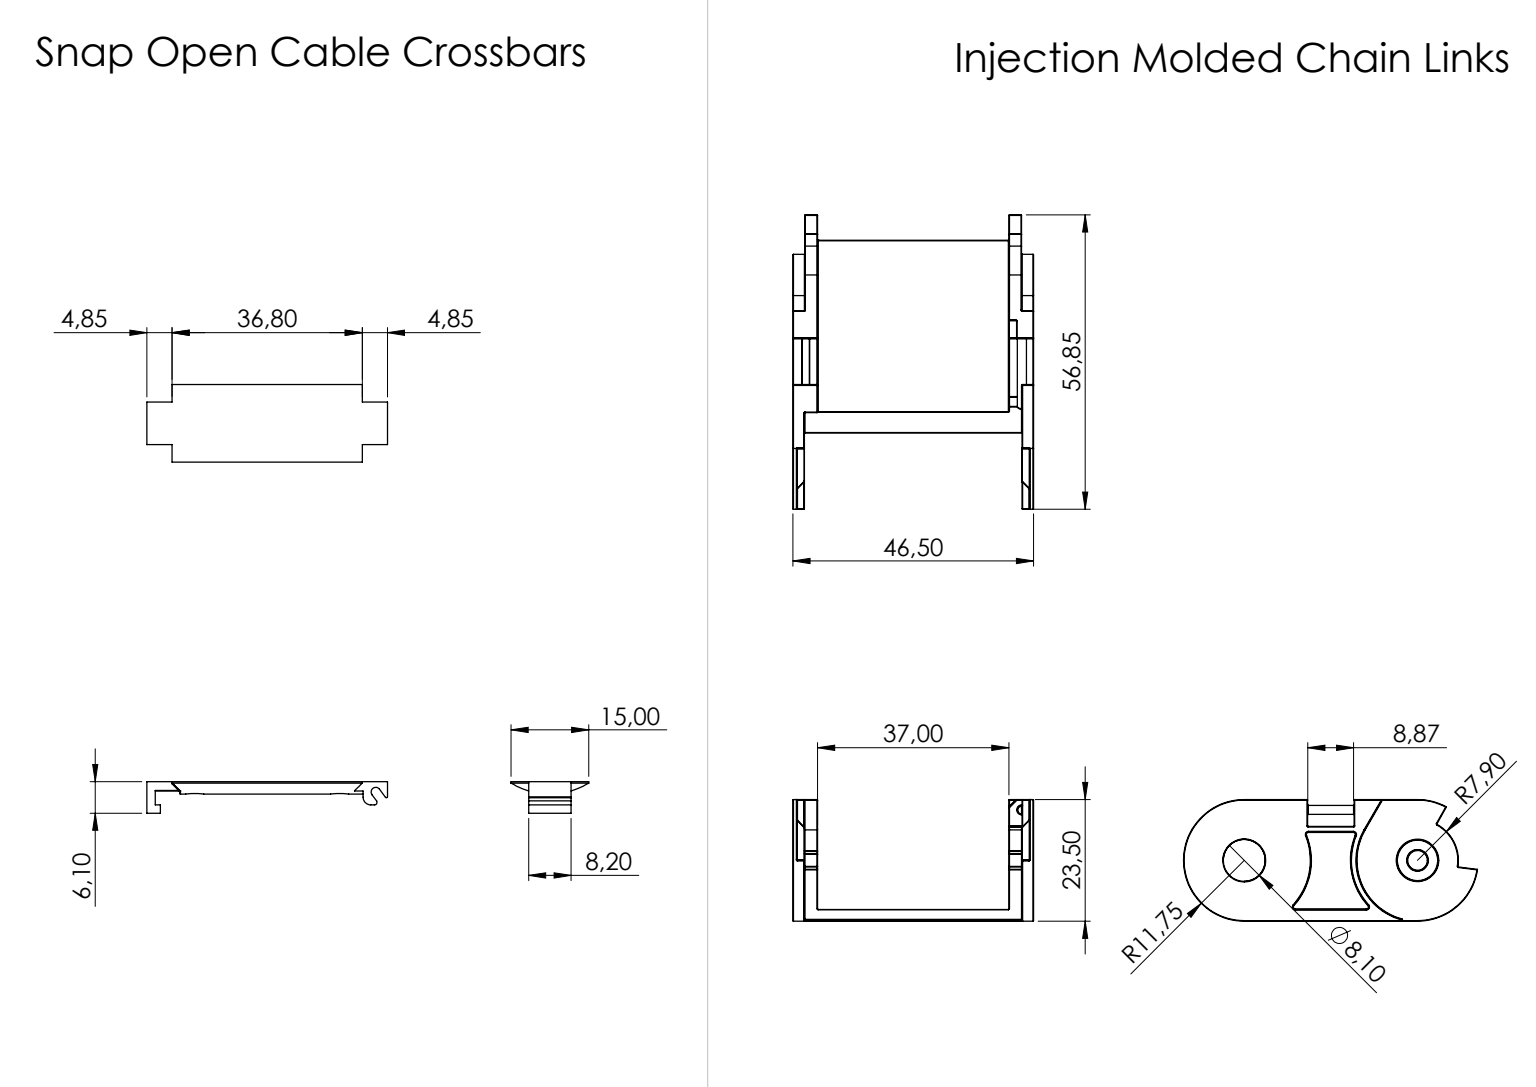
ISO-10303-21;
HEADER;
FILE_DESCRIPTION (('STEP AP214'),
    '1' );
FILE_NAME ('Snap Open Cable Crossbars.step',
    '2026-10-08T22:59:04',
    ( '' ),
    ( '' ),
    'SwSTEP 2.0',
    'SolidWorks 2020',
    '' );
FILE_SCHEMA (( 'AUTOMOTIVE_DESIGN' ));
ENDSEC;

DATA;
#1=CARTESIAN_POINT ( 'NONE',  ( -16.92989143108098204, 9.949999999999981526, -12.88248387475667656 ) ) ;
#36=CARTESIAN_POINT ( 'NONE',  ( -17.29838795458766043, 10.37154985795013218, -11.39525871738185714 ) ) ;
#202=CARTESIAN_POINT ( 'NONE',  ( 20.99999999999999645, 9.749999999999982236, -9.250000000000001776 ) ) ;
#413=CYLINDRICAL_SURFACE ( 'NONE', #45294, 1.749999999999998002 ) ;
#816=VERTEX_POINT ( 'NONE', #22856 ) ;
#827=FACE_OUTER_BOUND ( 'NONE', #190311, .T. ) ;
#850=CARTESIAN_POINT ( 'NONE',  ( -16.89797118371581419, 9.976380722644179855, -12.56270663244076857 ) ) ;
#880=FACE_OUTER_BOUND ( 'NONE', #179454, .T. ) ;
#1084=EDGE_CURVE ( 'NONE', #166202, #45065, #38658, .T. ) ;
#1259=CARTESIAN_POINT ( 'NONE',  ( -12.33960340485503515, 9.360749169915104417, -17.31457014060726962 ) ) ;
#1268=EDGE_CURVE ( 'NONE', #177395, #152802, #103725, .T. ) ;
#1311=DIRECTION ( 'NONE',  ( 1.000000000000000000, 0.000000000000000000, 0.000000000000000000 ) ) ;
#1354=ADVANCED_FACE ( 'NONE', ( #88580 ), #208179, .T. ) ;
#1447=DIRECTION ( 'NONE',  ( 1.652117596168391700E-15, 1.000000000000000000, -0.000000000000000000 ) ) ;
#1682=EDGE_CURVE ( 'NONE', #64185, #88756, #170443, .T. ) ;
#2076=AXIS2_PLACEMENT_3D ( 'NONE', #145577, #223822, #26957 ) ;
#2425=AXIS2_PLACEMENT_3D ( 'NONE', #153513, #135160, #16531 ) ;
#2428=ORIENTED_EDGE ( 'NONE', *, *, #175814, .F. ) ;
#2434=CARTESIAN_POINT ( 'NONE',  ( -16.94445028196807002, 9.992063609697737547, -20.89266982158155628 ) ) ;
#2476=APPLICATION_CONTEXT ( 'automotive_design' ) ;
#2634=CARTESIAN_POINT ( 'NONE',  ( -16.97683809663752186, 9.949999999999983302, -9.250000000000001776 ) ) ;
#2765=CARTESIAN_POINT ( 'NONE',  ( -17.78241384942186087, 10.85557575278904352, -23.25096232753543646 ) ) ;
#2813=EDGE_LOOP ( 'NONE', ( #157991, #36685, #88276, #78622 ) ) ;
#2957=FACE_OUTER_BOUND ( 'NONE', #112372, .T. ) ;
#3084=VECTOR ( 'NONE', #229687, 1000.000000000000000 ) ;
#3180=CARTESIAN_POINT ( 'NONE',  ( -16.80100914604134488, 9.943149094103565844, -20.81704412728764453 ) ) ;
#3672=ORIENTED_EDGE ( 'NONE', *, *, #139542, .F. ) ;
#4041=CARTESIAN_POINT ( 'NONE',  ( -12.47155713865592119, 9.375669526425772560, -15.86779000938594031 ) ) ;
#4143=DIRECTION ( 'NONE',  ( 1.186688945009009831E-16, -1.000000000000000000, 0.000000000000000000 ) ) ;
#4327=CARTESIAN_POINT ( 'NONE',  ( -23.25000000000000355, 5.649999999999983480, -12.65000000000000213 ) ) ;
#4347=FACE_OUTER_BOUND ( 'NONE', #98803, .T. ) ;
#4390=( BOUNDED_CURVE ( )  B_SPLINE_CURVE ( 3, ( #73328, #206387, #207681, #32928 ),
 .UNSPECIFIED., .F., .F. ) 
 B_SPLINE_CURVE_WITH_KNOTS ( ( 4, 4 ),
 ( 1.570796326794908992, 2.617993877991502849 ),
 .UNSPECIFIED. ) 
 CURVE ( )  GEOMETRIC_REPRESENTATION_ITEM ( )  RATIONAL_B_SPLINE_CURVE ( ( 1.000000000000000000, 0.9106836025229597675, 0.9106836025229597675, 1.000000000000000000 ) ) 
 REPRESENTATION_ITEM ( '' )  );
#4466=CARTESIAN_POINT ( 'NONE',  ( 14.22916352759893499, 9.457410930290162554, -18.49991590874628500 ) ) ;
#4575=CARTESIAN_POINT ( 'NONE',  ( -17.01825945287481545, 9.949999999999983302, -20.75000000000000000 ) ) ;
#4760=CARTESIAN_POINT ( 'NONE',  ( 18.39999999999999503, 11.74999999999998224, -20.85000000000000142 ) ) ;
#4794=( BOUNDED_SURFACE ( )  B_SPLINE_SURFACE ( 3, 2, ( 
 ( #64703, #180813, #239501 ),
 ( #179541, #850, #161255 ),
 ( #122121, #63409, #201646 ),
 ( #139068, #120862, #98653 ) ),
 .UNSPECIFIED., .F., .F., .T. ) 
 B_SPLINE_SURFACE_WITH_KNOTS ( ( 4, 4 ),
 ( 3, 3 ),
 ( 0.0008258556059633813742, 0.0009616864997632797044 ),
 ( 0.000000000000000000, 1.000000000000000000 ),
 .UNSPECIFIED. ) 
 GEOMETRIC_REPRESENTATION_ITEM ( )  RATIONAL_B_SPLINE_SURFACE ( (
 ( 1.000000000000000000, 0.9152888060719355234, 1.000000000000000000),
 ( 1.000000000000000000, 0.9327727094138189567, 1.000000000000000000),
 ( 1.000000000000000000, 0.9369023509258441740, 1.000000000000000000),
 ( 1.000000000000000000, 0.9246339933864472505, 1.000000000000000000) ) ) 
 REPRESENTATION_ITEM ( '' )  SURFACE ( )  );
#4866=CARTESIAN_POINT ( 'NONE',  ( -16.87331047859651179, 9.949999999999986855, -12.65000000000000213 ) ) ;
#4911=CARTESIAN_POINT ( 'NONE',  ( -16.94878442675511465, 9.991729102990998257, -20.88821957563787635 ) ) ;
#4939=VECTOR ( 'NONE', #199116, 1000.000000000000000 ) ;
#4994=DIRECTION ( 'NONE',  ( 1.000000000000000000, 0.000000000000000000, 0.000000000000000000 ) ) ;
#5134=AXIS2_PLACEMENT_3D ( 'NONE', #210609, #250995, #127226 ) ;
#5409=VERTEX_POINT ( 'NONE', #97085 ) ;
#5553=CARTESIAN_POINT ( 'NONE',  ( 20.73486653747088226, 7.250000000000026645, -12.65000000000000568 ) ) ;
#5607=CARTESIAN_POINT ( 'NONE',  ( -16.89208623190940273, 9.951577948975481647, -20.85527220321827002 ) ) ;
#6030=FACE_OUTER_BOUND ( 'NONE', #166234, .T. ) ;
#6408=CARTESIAN_POINT ( 'NONE',  ( -12.60829076262180060, 9.389529397466734650, -17.81710791289367535 ) ) ;
#6428=PLANE ( 'NONE',  #186510 ) ;
#6469=AXIS2_PLACEMENT_3D ( 'NONE', #223394, #44779, #100847 ) ;
#6649=AXIS2_PLACEMENT_3D ( 'NONE', #142927, #174758, #96432 ) ;
#6857=DIRECTION ( 'NONE',  ( 0.5932847527679299127, -0.8049926720990051576, 6.366092712777055223E-16 ) ) ;
#6912=( NAMED_UNIT ( * ) SI_UNIT ( $, .STERADIAN. ) SOLID_ANGLE_UNIT ( ) );
#6991=ORIENTED_EDGE ( 'NONE', *, *, #49751, .F. ) ;
#7235=VERTEX_POINT ( 'NONE', #177601 ) ;
#7280=ADVANCED_FACE ( 'NONE', ( #99288 ), #178892, .F. ) ;
#7551=CARTESIAN_POINT ( 'NONE',  ( -16.87036670365548474, 10.08494996325527460, -20.94999999999999929 ) ) ;
#7806=FACE_OUTER_BOUND ( 'NONE', #23507, .T. ) ;
#7861=AXIS2_PLACEMENT_3D ( 'NONE', #232656, #11018, #53993 ) ;
#7969=VERTEX_POINT ( 'NONE', #147105 ) ;
#8041=DIRECTION ( 'NONE',  ( 0.000000000000000000, 0.000000000000000000, -1.000000000000000000 ) ) ;
#8080=DIRECTION ( 'NONE',  ( 1.000000000000000000, 0.000000000000000000, -0.000000000000000000 ) ) ;
#8152=ADVANCED_FACE ( 'NONE', ( #23040 ), #4794, .T. ) ;
#8294=CARTESIAN_POINT ( 'NONE',  ( -23.25000000000000355, 5.649999999999983480, -9.250000000000001776 ) ) ;
#8359=LINE ( 'NONE', #9625, #132434 ) ;
#8639=CARTESIAN_POINT ( 'NONE',  ( -16.93658623642901162, 9.980381671657131193, -12.61190272912918964 ) ) ;
#8647=FACE_OUTER_BOUND ( 'NONE', #161256, .T. ) ;
#8875=CARTESIAN_POINT ( 'NONE',  ( -16.86578989773640913, 9.984809801258796469, -20.96466488662223426 ) ) ;
#9058=AXIS2_PLACEMENT_3D ( 'NONE', #124611, #201562, #162464 ) ;
#9153=DIRECTION ( 'NONE',  ( 1.000000000000000000, -0.000000000000000000, -0.000000000000000000 ) ) ;
#9473=ORIENTED_EDGE ( 'NONE', *, *, #1084, .F. ) ;
#9625=CARTESIAN_POINT ( 'NONE',  ( -23.25000000000000355, 11.74999999999998224, -24.25000000000000000 ) ) ;
#9635=DIRECTION ( 'NONE',  ( -1.020425574104004196E-15, 0.000000000000000000, -1.000000000000000000 ) ) ;
#9814=DIRECTION ( 'NONE',  ( 0.000000000000000000, 1.000000000000000000, 3.662759245464225434E-15 ) ) ;
#9888=FACE_OUTER_BOUND ( 'NONE', #185101, .T. ) ;
#10255=CARTESIAN_POINT ( 'NONE',  ( -16.93226657140833069, 9.999543822724415776, -12.57871311097362188 ) ) ;
#10281=CARTESIAN_POINT ( 'NONE',  ( -15.51798037960205257, 9.376659938533535410, -17.62819254821728876 ) ) ;
#10503=CARTESIAN_POINT ( 'NONE',  ( -18.40000000000000213, 11.47316190336247388, -12.65000000000000213 ) ) ;
#10606=CARTESIAN_POINT ( 'NONE',  ( -17.11825945287482753, 10.04999999999998295, -12.65000000000000213 ) ) ;
#10621=ORIENTED_EDGE ( 'NONE', *, *, #251969, .F. ) ;
#10937=DIRECTION ( 'NONE',  ( 1.000000000000000000, 0.000000000000000000, -1.020425574104004196E-15 ) ) ;
#10962=CARTESIAN_POINT ( 'NONE',  ( -16.86133551771149541, 9.949999999999983302, -20.80134343454665213 ) ) ;
#10978=ORIENTED_EDGE ( 'NONE', *, *, #1268, .F. ) ;
#11018=DIRECTION ( 'NONE',  ( 1.186688945009009831E-16, -1.000000000000000000, 0.000000000000000000 ) ) ;
#11145=CYLINDRICAL_SURFACE ( 'NONE', #172793, 0.1999999999999987899 ) ;
#11416=VECTOR ( 'NONE', #214106, 1000.000000000000000 ) ;
#11464=ORIENTED_EDGE ( 'NONE', *, *, #189871, .T. ) ;
#11901=LINE ( 'NONE', #189239, #247679 ) ;
#11925=AXIS2_PLACEMENT_3D ( 'NONE', #48197, #126453, #143448 ) ;
#12016=LINE ( 'NONE', #69418, #173208 ) ;
#12179=( BOUNDED_CURVE ( )  B_SPLINE_CURVE ( 3, ( #253467, #111406, #110112, #74881 ),
 .UNSPECIFIED., .F., .T. ) 
 B_SPLINE_CURVE_WITH_KNOTS ( ( 4, 4 ),
 ( 0.3000847527772381174, 0.5497968875596821459 ),
 .UNSPECIFIED. ) 
 CURVE ( )  GEOMETRIC_REPRESENTATION_ITEM ( )  RATIONAL_B_SPLINE_CURVE ( ( 1.000000000000000000, 0.9948104011409419911, 0.9948104011409419911, 1.000000000000000000 ) ) 
 REPRESENTATION_ITEM ( '' )  );
#12209=CARTESIAN_POINT ( 'NONE',  ( 13.22461703343584638, 9.436662931799084220, -18.32303673229488794 ) ) ;
#12294=CARTESIAN_POINT ( 'NONE',  ( 18.39999999999999503, 11.74999999999998224, -12.65000000000000213 ) ) ;
#12434=FACE_OUTER_BOUND ( 'NONE', #157664, .T. ) ;
#12804=DIRECTION ( 'NONE',  ( -1.000000000000000000, 1.652117596168391700E-15, 0.000000000000000000 ) ) ;
#12859=VECTOR ( 'NONE', #213521, 1000.000000000000000 ) ;
#12920=VERTEX_POINT ( 'NONE', #158155 ) ;
#12996=EDGE_LOOP ( 'NONE', ( #33480, #208453, #194883, #57495 ) ) ;
#13020=EDGE_CURVE ( 'NONE', #33881, #237173, #25040, .T. ) ;
#13083=VECTOR ( 'NONE', #54298, 1000.000000000000000 ) ;
#13218=DIRECTION ( 'NONE',  ( -0.5932847527679310229, 0.8049926720990042694, -6.366092712777067056E-16 ) ) ;
#13289=VECTOR ( 'NONE', #57030, 1000.000000000000000 ) ;
#13474=CARTESIAN_POINT ( 'NONE',  ( -16.77431908686106610, 9.945805754517978770, -12.66416078234975373 ) ) ;
#13481=CARTESIAN_POINT ( 'NONE',  ( 13.12229106158772929, 9.430637101696738966, -18.26826061806094614 ) ) ;
#13689=CARTESIAN_POINT ( 'NONE',  ( 12.25000000000000000, 9.349999999999983658, -16.74999999999999645 ) ) ;
#13778=FACE_OUTER_BOUND ( 'NONE', #117729, .T. ) ;
#13843=DIRECTION ( 'NONE',  ( -1.000000000000000000, 0.000000000000000000, -0.000000000000000000 ) ) ;
#13882=VECTOR ( 'NONE', #129686, 1000.000000000000000 ) ;
#14008=( LENGTH_UNIT ( ) NAMED_UNIT ( * ) SI_UNIT ( .MILLI., .METRE. ) );
#14057=AXIS2_PLACEMENT_3D ( 'NONE', #196592, #214877, #97468 ) ;
#14206=CARTESIAN_POINT ( 'NONE',  ( 20.73486653747090003, 7.250000000000026645, -20.85000000000000142 ) ) ;
#14615=VERTEX_POINT ( 'NONE', #34702 ) ;
#14701=ORIENTED_EDGE ( 'NONE', *, *, #49751, .T. ) ;
#14727=CARTESIAN_POINT ( 'NONE',  ( -16.94275863006528482, 9.989496048667513506, -20.89169738207657900 ) ) ;
#14735=CARTESIAN_POINT ( 'NONE',  ( -16.77683809663752257, 23.65833333333332433, -16.75000000000000000 ) ) ;
#15047=CARTESIAN_POINT ( 'NONE',  ( -18.35235881385853318, 11.47341900771289502, -9.250000000000001776 ) ) ;
#15165=PLANE ( 'NONE',  #223421 ) ;
#15643=ADVANCED_FACE ( 'NONE', ( #217183 ), #15165, .T. ) ;
#15874=ORIENTED_EDGE ( 'NONE', *, *, #175580, .T. ) ;
#15938=CARTESIAN_POINT ( 'NONE',  ( 23.04999999999999716, 8.822561741666397950, -12.65000000000000746 ) ) ;
#15952=CYLINDRICAL_SURFACE ( 'NONE', #238205, 0.1000000000000001443 ) ;
#16009=CARTESIAN_POINT ( 'NONE',  ( -16.93301857435212554, 9.976309354735457546, -20.88577557116142813 ) ) ;
#16028=CARTESIAN_POINT ( 'NONE',  ( -16.87036670365548474, 9.989418819301645769, -20.97956011730205006 ) ) ;
#16220=DIRECTION ( 'NONE',  ( -1.000000000000000000, -0.000000000000000000, 1.073024830501117725E-15 ) ) ;
#16242=CIRCLE ( 'NONE', #7861, 1.749999999999998002 ) ;
#16369=VECTOR ( 'NONE', #222084, 1000.000000000000000 ) ;
#16512=CARTESIAN_POINT ( 'NONE',  ( -16.93826681692523195, 10.01142872028771258, -20.94545846735944039 ) ) ;
#16531=DIRECTION ( 'NONE',  ( 1.000000000000000000, 0.000000000000000000, 0.000000000000000000 ) ) ;
#16707=EDGE_CURVE ( 'NONE', #101212, #219433, #149599, .T. ) ;
#16728=EDGE_LOOP ( 'NONE', ( #255760, #202446, #84176, #145665, #190088, #218155 ) ) ;
#16867=VECTOR ( 'NONE', #108313, 1000.000000000000000 ) ;
#16914=ORIENTED_EDGE ( 'NONE', *, *, #147422, .F. ) ;
#17161=VERTEX_POINT ( 'NONE', #4327 ) ;
#17354=CARTESIAN_POINT ( 'NONE',  ( -16.77683809663752257, 9.945835743204147761, -20.83605098089580210 ) ) ;
#17399=EDGE_CURVE ( 'NONE', #195135, #51112, #36791, .T. ) ;
#17460=( BOUNDED_CURVE ( )  B_SPLINE_CURVE ( 3, ( #10606, #90112, #169715, #191834 ),
 .UNSPECIFIED., .F., .F. ) 
 B_SPLINE_CURVE_WITH_KNOTS ( ( 4, 4 ),
 ( 4.712388980384689674, 5.672655318024675708 ),
 .UNSPECIFIED. ) 
 CURVE ( )  GEOMETRIC_REPRESENTATION_ITEM ( )  RATIONAL_B_SPLINE_CURVE ( ( 1.000000000000000000, 0.9246222802177378464, 0.9246222802177378464, 1.000000000000000000 ) ) 
 REPRESENTATION_ITEM ( '' )  );
#17529=CARTESIAN_POINT ( 'NONE',  ( 14.56326696814971555, 9.446648990628860432, -15.08916329592317851 ) ) ;
#17932=DIRECTION ( 'NONE',  ( -1.186688945009010077E-16, 1.000000000000000000, 0.000000000000000000 ) ) ;
#17968=CARTESIAN_POINT ( 'NONE',  ( -20.65000000000000568, 7.249999999999983125, -9.250000000000001776 ) ) ;
#18030=VERTEX_POINT ( 'NONE', #147078 ) ;
#18241=PRODUCT_CONTEXT ( 'NONE', #208885, 'mechanical' ) ;
#18310=CARTESIAN_POINT ( 'NONE',  ( -23.25000000000000355, 5.649999999999983480, -9.250000000000001776 ) ) ;
#18323=FACE_OUTER_BOUND ( 'NONE', #43596, .T. ) ;
#18823=CARTESIAN_POINT ( 'NONE',  ( 15.74999999999999645, 9.349999999999983658, -16.75000000000000000 ) ) ;
#18974=CARTESIAN_POINT ( 'NONE',  ( -18.40000000000000213, 5.649999999999983480, -12.65000000000000213 ) ) ;
#19226=DIRECTION ( 'NONE',  ( 1.000000000000000000, 1.186688945009010077E-16, 0.000000000000000000 ) ) ;
#19555=LINE ( 'NONE', #219015, #142994 ) ;
#19583=ORIENTED_EDGE ( 'NONE', *, *, #49360, .F. ) ;
#19621=CARTESIAN_POINT ( 'NONE',  ( -17.22767730082987825, 10.34924421246758719, -11.35757130942880977 ) ) ;
#19659=EDGE_LOOP ( 'NONE', ( #155323, #54902, #200500, #42750 ) ) ;
#19983=AXIS2_PLACEMENT_3D ( 'NONE', #126963, #206498, #82661 ) ;
#20072=CARTESIAN_POINT ( 'NONE',  ( -23.25000000000000355, 11.74999999999998224, -12.65000000000000213 ) ) ;
#20073=SURFACE_STYLE_FILL_AREA ( #120478 ) ;
#20155=ADVANCED_FACE ( 'NONE', ( #147502 ), #167102, .F. ) ;
#20208=CARTESIAN_POINT ( 'NONE',  ( -16.87683809663752044, 9.864913447280185821, -20.22428155130396021 ) ) ;
#20381=ORIENTED_EDGE ( 'NONE', *, *, #229317, .F. ) ;
#20491=FACE_OUTER_BOUND ( 'NONE', #166229, .T. ) ;
#20500=AXIS2_PLACEMENT_3D ( 'NONE', #162836, #4994, #63705 ) ;
#20521=ORIENTED_EDGE ( 'NONE', *, *, #17399, .F. ) ;
#20595=EDGE_CURVE ( 'NONE', #35963, #143544, #181618, .T. ) ;
#21033=CARTESIAN_POINT ( 'NONE',  ( -16.97683809663752186, 9.949999999999983302, -13.40236401819648648 ) ) ;
#21051=CARTESIAN_POINT ( 'NONE',  ( -21.64999999999999858, 9.349999999999978328, -20.85000000000000142 ) ) ;
#21147=CARTESIAN_POINT ( 'NONE',  ( -33.72168855820452649, 11.47316190336247033, -9.249999999999998224 ) ) ;
#21154=EDGE_CURVE ( 'NONE', #7969, #237173, #245177, .T. ) ;
#21199=VECTOR ( 'NONE', #124420, 1000.000000000000000 ) ;
#21286=ORIENTED_EDGE ( 'NONE', *, *, #159207, .F. ) ;
#21319=PLANE ( 'NONE',  #241824 ) ;
#21353=EDGE_CURVE ( 'NONE', #101212, #222175, #16242, .T. ) ;
#21382=EDGE_CURVE ( 'NONE', #60760, #177395, #12179, .T. ) ;
#21496=CARTESIAN_POINT ( 'NONE',  ( -16.88705144915421030, 9.949999999999981526, -20.56902140528771739 ) ) ;
#21501=CARTESIAN_POINT ( 'NONE',  ( -16.81453563122428818, 9.939100205436954383, -20.78825866064531880 ) ) ;
#21515=CARTESIAN_POINT ( 'NONE',  ( 18.39999999999999503, 11.74999999999998224, -20.85000000000000142 ) ) ;
#21775=DIRECTION ( 'NONE',  ( -0.7071067811865487940, 0.7071067811865463515, 0.000000000000000000 ) ) ;
#21962=EDGE_LOOP ( 'NONE', ( #16914, #90521, #72160, #246736 ) ) ;
#22093=CARTESIAN_POINT ( 'NONE',  ( 20.99999999999999645, 9.749999999999982236, -12.65000000000000568 ) ) ;
#22353=CARTESIAN_POINT ( 'NONE',  ( -12.84409460144754433, 9.410682294267951775, -15.43114344194827581 ) ) ;
#22370=CARTESIAN_POINT ( 'NONE',  ( -16.91256925476569961, 9.985731158128169582, -20.96764248900526439 ) ) ;
#22621=B_SPLINE_CURVE_WITH_KNOTS ( 'NONE', 3,
 ( #154744, #16512, #93447, #173048, #153491, #135134, #36070, #232999, #214684, #195162, #96013, #255032, #129999, #209563, #30956, #170489 ),
 .UNSPECIFIED., .F., .F.,
 ( 4, 3, 3, 3, 3, 4 ),
 ( 0.000000000000000000, 1.810570668010556722E-05, 2.740575833571567380E-05, 4.256816319435758028E-05, 5.213463471025523268E-05, 6.641585710718234082E-05 ),
 .UNSPECIFIED. ) ;
#22712=( BOUNDED_CURVE ( )  B_SPLINE_CURVE ( 3, ( #227470, #48840, #207945, #192227 ),
 .UNSPECIFIED., .F., .F. ) 
 B_SPLINE_CURVE_WITH_KNOTS ( ( 4, 4 ),
 ( 1.570796326794885012, 3.141592653589794448 ),
 .UNSPECIFIED. ) 
 CURVE ( )  GEOMETRIC_REPRESENTATION_ITEM ( )  RATIONAL_B_SPLINE_CURVE ( ( 1.000000000000000000, 0.8047378541243619399, 0.8047378541243619399, 1.000000000000000000 ) ) 
 REPRESENTATION_ITEM ( '' )  );
#22727=EDGE_CURVE ( 'NONE', #203977, #5409, #248862, .T. ) ;
#22788=CARTESIAN_POINT ( 'NONE',  ( -16.84793658983420173, 9.949999999999983302, -20.76635332218982910 ) ) ;
#22795=CARTESIAN_POINT ( 'NONE',  ( -16.80469485234340610, 9.942151663141038043, -20.80996684393117135 ) ) ;
#22856=CARTESIAN_POINT ( 'NONE',  ( -17.11825945287482753, 10.04999999999998295, -12.65000000000000213 ) ) ;
#23040=FACE_OUTER_BOUND ( 'NONE', #19659, .T. ) ;
#23258=CARTESIAN_POINT ( 'NONE',  ( -20.65000000000000568, 5.649999999999983480, -9.250000000000001776 ) ) ;
#23445=CARTESIAN_POINT ( 'NONE',  ( -14.77538296656415184, 9.436662931799085996, -18.32303673229489149 ) ) ;
#23507=EDGE_LOOP ( 'NONE', ( #57717, #253160, #179128, #59181 ) ) ;
#23649=CARTESIAN_POINT ( 'NONE',  ( -15.06774609480955363, 9.417651958841000592, -15.35878739244043345 ) ) ;
#23659=CARTESIAN_POINT ( 'NONE',  ( 18.39999999999999147, 8.822561741666397950, -9.250000000000001776 ) ) ;
#23666=CARTESIAN_POINT ( 'NONE',  ( -18.41431012584568805, 11.48747202920817223, -24.27323601310168399 ) ) ;
#23835=ORIENTED_EDGE ( 'NONE', *, *, #81866, .F. ) ;
#23843=CARTESIAN_POINT ( 'NONE',  ( -23.25000000000000355, 5.649999999999983480, -20.85000000000000142 ) ) ;
#23960=PLANE ( 'NONE',  #112128 ) ;
#24301=CARTESIAN_POINT ( 'NONE',  ( -16.87036670365549895, 10.08494996325527460, -12.55000000000000249 ) ) ;
#24387=DIRECTION ( 'NONE',  ( 1.000000000000000000, -0.000000000000000000, -0.000000000000000000 ) ) ;
#24490=CARTESIAN_POINT ( 'NONE',  ( -16.89060415895971090, 9.951220762802197584, -12.64592022427046203 ) ) ;
#24938=EDGE_CURVE ( 'NONE', #187424, #206683, #225373, .T. ) ;
#25035=EDGE_CURVE ( 'NONE', #195135, #201670, #188355, .T. ) ;
#25040=LINE ( 'NONE', #182832, #147141 ) ;
#25053=DIRECTION ( 'NONE',  ( 1.000000000000000000, 0.000000000000000000, -0.000000000000000000 ) ) ;
#25524=ORIENTED_EDGE ( 'NONE', *, *, #180090, .T. ) ;
#25572=CARTESIAN_POINT ( 'NONE',  ( 20.73486653747088937, 7.750000000000025757, -9.250000000000001776 ) ) ;
#25783=CYLINDRICAL_SURFACE ( 'NONE', #213675, 1.500000000000001332 ) ;
#25802=ORIENTED_EDGE ( 'NONE', *, *, #247500, .T. ) ;
#25834=DIRECTION ( 'NONE',  ( 1.000000000000000000, -0.000000000000000000, -0.000000000000000000 ) ) ;
#25989=CARTESIAN_POINT ( 'NONE',  ( -12.30589683808040391, 9.356746017078247490, -17.20335972136419400 ) ) ;
#26607=CARTESIAN_POINT ( 'NONE',  ( -15.75000000000000355, 9.849999999999978328, -16.75000000000000355 ) ) ;
#26839=CARTESIAN_POINT ( 'NONE',  ( -17.29158576265543346, 10.36474766601791586, -22.08275824479217775 ) ) ;
#26957=DIRECTION ( 'NONE',  ( 0.000000000000000000, 0.000000000000000000, 1.000000000000000000 ) ) ;
#27150=CARTESIAN_POINT ( 'NONE',  ( 20.73486653747088582, 7.250000000000026645, -9.250000000000001776 ) ) ;
#27284=FACE_BOUND ( 'NONE', #27743, .T. ) ;
#27305=VECTOR ( 'NONE', #238398, 1000.000000000000000 ) ;
#27497=VECTOR ( 'NONE', #66820, 1000.000000000000000 ) ;
#27743=EDGE_LOOP ( 'NONE', ( #45441, #134007 ) ) ;
#27882=ADVANCED_FACE ( 'NONE', ( #30508 ), #188274, .F. ) ;
#27978=VERTEX_POINT ( 'NONE', #17354 ) ;
#28030=( BOUNDED_SURFACE ( )  B_SPLINE_SURFACE ( 3, 2, ( 
 ( #249522, #52578, #33078 ),
 ( #173875, #53880, #74764 ),
 ( #55123, #154311, #168742 ),
 ( #70901, #134672, #209094 ),
 ( #248228, #69603, #149146 ),
 ( #229942, #228680, #91719 ),
 ( #30478, #112577, #252071 ),
 ( #51271, #250784, #31779 ),
 ( #111287, #171311, #151725 ),
 ( #231252, #192126, #13474 ) ),
 .UNSPECIFIED., .F., .F., .F. ) 
 B_SPLINE_SURFACE_WITH_KNOTS ( ( 4, 2, 2, 2, 4 ),
 ( 3, 3 ),
 ( 0.002161241639767788603, 0.002579950749617449836, 0.002789305304542280452, 0.002893982582004695978, 0.002998659859467111069 ),
 ( 0.000000000000000000, 1.000000000000000000 ),
 .UNSPECIFIED. ) 
 GEOMETRIC_REPRESENTATION_ITEM ( )  RATIONAL_B_SPLINE_SURFACE ( (
 ( 1.000000000000000000, 0.7071067811864800712, 1.000000000000000000),
 ( 1.000000000000000000, 0.7632447400664645887, 1.000000000000000000),
 ( 1.000000000000000000, 0.8158073005108372744, 1.000000000000000000),
 ( 1.000000000000000000, 0.8906973462396270413, 1.000000000000000000),
 ( 1.000000000000000000, 0.9149408947800815595, 1.000000000000000000),
 ( 1.000000000000000000, 0.9493368785275272392, 1.000000000000000000),
 ( 1.000000000000000000, 0.9605194247156589871, 1.000000000000000000),
 ( 1.000000000000000000, 0.9803630264781161285, 1.000000000000000000),
 ( 1.000000000000000000, 0.9900844824271106681, 1.000000000000000000),
 ( 1.000000000000000000, 0.9894588281429282928, 1.000000000000000000) ) ) 
 REPRESENTATION_ITEM ( '' )  SURFACE ( )  );
#28151=PLANE ( 'NONE',  #5134 ) ;
#28343=PLANE ( 'NONE',  #214509 ) ;
#28391=DIRECTION ( 'NONE',  ( -0.000000000000000000, -0.000000000000000000, -1.000000000000000000 ) ) ;
#28480=CARTESIAN_POINT ( 'NONE',  ( -16.86337532320260735, 9.979967204224358568, -20.94892446898280980 ) ) ;
#28482=CYLINDRICAL_SURFACE ( 'NONE', #20500, 0.09999999999999939493 ) ;
#28535=VECTOR ( 'NONE', #219008, 1000.000000000000000 ) ;
#28727=EDGE_CURVE ( 'NONE', #184131, #86042, #85956, .T. ) ;
#28914=VECTOR ( 'NONE', #211018, 999.9999999999998863 ) ;
#28990=VERTEX_POINT ( 'NONE', #206590 ) ;
#29224=CARTESIAN_POINT ( 'NONE',  ( 15.31784899511109721, 9.396630376317714806, -17.90705739281830589 ) ) ;
#29249=CARTESIAN_POINT ( 'NONE',  ( -18.40000000000000213, 5.649999999999983480, -12.65000000000000213 ) ) ;
#29270=ORIENTED_EDGE ( 'NONE', *, *, #21154, .F. ) ;
#29462=CARTESIAN_POINT ( 'NONE',  ( 13.99999999999999822, 9.849999999999981881, -16.74999999999999645 ) ) ;
#29712=DIRECTION ( 'NONE',  ( -0.000000000000000000, -0.000000000000000000, -1.000000000000000000 ) ) ;
#29737=EDGE_CURVE ( 'NONE', #109071, #191176, #181304, .T. ) ;
#29931=ORIENTED_EDGE ( 'NONE', *, *, #35996, .T. ) ;
#30247=VECTOR ( 'NONE', #92407, 1000.000000000000000 ) ;
#30478=CARTESIAN_POINT ( 'NONE',  ( -16.87401514999235630, 9.949999999999983302, -12.71998200746783780 ) ) ;
#30485=CARTESIAN_POINT ( 'NONE',  ( -16.77180007708460963, 9.949999999999983302, -20.86438588104518388 ) ) ;
#30508=FACE_OUTER_BOUND ( 'NONE', #227736, .T. ) ;
#30956=CARTESIAN_POINT ( 'NONE',  ( -16.94132844910801694, 9.992436755180344576, -20.89620175598231455 ) ) ;
#31003=ORIENTED_EDGE ( 'NONE', *, *, #159207, .T. ) ;
#31041=CARTESIAN_POINT ( 'NONE',  ( -16.86420534634261514, 9.970615445591718640, -20.91833654923738806 ) ) ;
#31064=CARTESIAN_POINT ( 'NONE',  ( -16.77683809663752257, 9.949999999999983302, -20.85000000000000142 ) ) ;
#31779=CARTESIAN_POINT ( 'NONE',  ( -16.80621392010906945, 9.942202577507719852, -12.68959196541704060 ) ) ;
#31835=CARTESIAN_POINT ( 'NONE',  ( -16.97683809663752186, 9.949999999999983302, -20.09763598180368405 ) ) ;
#31863=LINE ( 'NONE', #12294, #204867 ) ;
#32013=DIRECTION ( 'NONE',  ( -1.000000000000000000, 0.000000000000000000, 0.000000000000000000 ) ) ;
#32597=CIRCLE ( 'NONE', #86689, 1.749999999999999778 ) ;
#32808=CARTESIAN_POINT ( 'NONE',  ( 20.27550659511089037, 9.216043722508839409, -20.85000000000000142 ) ) ;
#32836=VECTOR ( 'NONE', #178947, 1000.000000000000000 ) ;
#32846=EDGE_CURVE ( 'NONE', #140173, #47344, #174568, .T. ) ;
#32855=ORIENTED_EDGE ( 'NONE', *, *, #46103, .F. ) ;
#32863=ORIENTED_EDGE ( 'NONE', *, *, #139800, .F. ) ;
#32911=CARTESIAN_POINT ( 'NONE',  ( -15.55912972643740488, 8.490870273562565629, -20.85000000000000142 ) ) ;
#32928=CARTESIAN_POINT ( 'NONE',  ( -16.87331047859649757, 9.949999999999983302, -20.85000000000000142 ) ) ;
#32958=DIRECTION ( 'NONE',  ( 0.7071067811865463515, -0.7071067811865487940, 0.000000000000000000 ) ) ;
#33016=CARTESIAN_POINT ( 'NONE',  ( -17.04295772865485148, 10.02489942525999567, -20.85000000000000142 ) ) ;
#33078=CARTESIAN_POINT ( 'NONE',  ( -16.87683809663752399, 9.849999999999964118, -13.40236401819648115 ) ) ;
#33275=CARTESIAN_POINT ( 'NONE',  ( -16.87683809663752399, 23.65833333333332433, -16.75000000000000000 ) ) ;
#33326=DIRECTION ( 'NONE',  ( -0.000000000000000000, -0.000000000000000000, -1.000000000000000000 ) ) ;
#33379=DIRECTION ( 'NONE',  ( 0.000000000000000000, 0.000000000000000000, 1.000000000000000000 ) ) ;
#33480=ORIENTED_EDGE ( 'NONE', *, *, #182872, .T. ) ;
#33583=CARTESIAN_POINT ( 'NONE',  ( -21.65000000000000213, 7.249999999999983125, -20.85000000000000142 ) ) ;
#33644=DIRECTION ( 'NONE',  ( -1.000000000000000000, 0.000000000000000000, 0.000000000000000000 ) ) ;
#33881=VERTEX_POINT ( 'NONE', #38907 ) ;
#34232=ORIENTED_EDGE ( 'NONE', *, *, #81714, .F. ) ;
#34413=CARTESIAN_POINT ( 'NONE',  ( 20.99999999999999645, 9.749999999999982236, -20.84999999999999787 ) ) ;
#34561=CARTESIAN_POINT ( 'NONE',  ( 15.52844286134407703, 9.375669526425774336, -15.86779000938593676 ) ) ;
#34650=DIRECTION ( 'NONE',  ( -1.073024830501117725E-15, -0.000000000000000000, -1.000000000000000000 ) ) ;
#34702=CARTESIAN_POINT ( 'NONE',  ( 22.88900146558018989, 8.703904791112817563, -20.84999999999999432 ) ) ;
#34847=CARTESIAN_POINT ( 'NONE',  ( -18.40000000000000213, 11.74999999999998224, -12.65000000000000213 ) ) ;
#34943=CARTESIAN_POINT ( 'NONE',  ( -21.64999999999999858, 10.04999999999998295, -12.75000000000000178 ) ) ;
#35085=CARTESIAN_POINT ( 'NONE',  ( -17.04295772865479819, 10.02489942525997257, -12.65000000000000391 ) ) ;
#35378=ORIENTED_EDGE ( 'NONE', *, *, #180100, .F. ) ;
#35502=ORIENTED_EDGE ( 'NONE', *, *, #85243, .F. ) ;
#35911=ORIENTED_EDGE ( 'NONE', *, *, #141580, .T. ) ;
#35963=VERTEX_POINT ( 'NONE', #122065 ) ;
#35996=EDGE_CURVE ( 'NONE', #45065, #83518, #81694, .T. ) ;
#36004=ORIENTED_EDGE ( 'NONE', *, *, #123280, .F. ) ;
#36053=EDGE_LOOP ( 'NONE', ( #209141, #99369 ) ) ;
#36070=CARTESIAN_POINT ( 'NONE',  ( -16.93262454970419384, 10.00202046793035748, -20.92707622623731467 ) ) ;
#36403=ORIENTED_EDGE ( 'NONE', *, *, #193056, .T. ) ;
#36562=VECTOR ( 'NONE', #33326, 1000.000000000000000 ) ;
#36592=VECTOR ( 'NONE', #50443, 1000.000000000000000 ) ;
#36685=ORIENTED_EDGE ( 'NONE', *, *, #99249, .T. ) ;
#36791=LINE ( 'NONE', #116305, #11416 ) ;
#36866=LINE ( 'NONE', #21147, #32836 ) ;
#37305=CARTESIAN_POINT ( 'NONE',  ( 17.74533788810830615, 10.81849979147079210, -10.31362267494758100 ) ) ;
#37678=EDGE_CURVE ( 'NONE', #212402, #50885, #211616, .T. ) ;
#37882=CARTESIAN_POINT ( 'NONE',  ( -16.89020380669787258, 9.949999999999985079, -12.75741114811056853 ) ) ;
#38000=ORIENTED_EDGE ( 'NONE', *, *, #83123, .F. ) ;
#38023=PLANE ( 'NONE',  #247973 ) ;
#38038=ADVANCED_FACE ( 'NONE', ( #147474 ), #44132, .T. ) ;
#38110=ORIENTED_EDGE ( 'NONE', *, *, #71892, .F. ) ;
#38113=AXIS2_PLACEMENT_3D ( 'NONE', #123784, #202036, #142048 ) ;
#38219=DIRECTION ( 'NONE',  ( 0.000000000000000000, -1.000000000000000000, 0.000000000000000000 ) ) ;
#38280=FACE_OUTER_BOUND ( 'NONE', #72906, .T. ) ;
#38335=CARTESIAN_POINT ( 'NONE',  ( -16.87845715379269507, 9.957858113897010810, -12.62380065105889493 ) ) ;
#38353=CARTESIAN_POINT ( 'NONE',  ( -16.88593481969334320, 9.950560090084310971, -20.85187225694449609 ) ) ;
#38396=CARTESIAN_POINT ( 'NONE',  ( 15.70340296795548518, 9.355888454502546026, -16.28864289677800059 ) ) ;
#38480=ORIENTED_EDGE ( 'NONE', *, *, #90094, .F. ) ;
#38658=B_SPLINE_CURVE_WITH_KNOTS ( 'NONE', 3,
 ( #255634, #238687, #137022, #216553 ),
 .UNSPECIFIED., .F., .F.,
 ( 4, 4 ),
 ( 0.000000000000000000, 7.713889350927971339E-05 ),
 .UNSPECIFIED. ) ;
#38907=CARTESIAN_POINT ( 'NONE',  ( 20.09999999999999787, 9.749999999999982236, -12.65000000000000391 ) ) ;
#38908=CARTESIAN_POINT ( 'NONE',  ( -16.97092634996667471, 10.00088896634854052, -12.63014276629761135 ) ) ;
#38931=LINE ( 'NONE', #196698, #27305 ) ;
#39167=CARTESIAN_POINT ( 'NONE',  ( -16.86132326855786090, 9.949999999999983302, -12.69863578466831910 ) ) ;
#39184=CARTESIAN_POINT ( 'NONE',  ( -16.94445028196808778, 9.992063609697733995, -12.60733017841845438 ) ) ;
#39456=EDGE_CURVE ( 'NONE', #222175, #140980, #19555, .T. ) ;
#39471=B_SPLINE_CURVE_WITH_KNOTS ( 'NONE', 3,
 ( #161864, #167014, #246505, #202253, #45739, #224371, #23649, #204797, #220537, #125286, #41919, #121462, #122735, #64023, #84830, #43183, #200963, #243933, #103129, #182704, #22353, #83552, #4041, #181424, #62744, #142269 ),
 .UNSPECIFIED., .F., .F.,
 ( 4, 2, 2, 2, 2, 2, 2, 2, 2, 2, 2, 2, 4 ),
 ( 0.005476422646581358654, 0.006160811967703566129, 0.006845201288825772737, 0.007187395949386878209, 0.007529590609947983681, 0.007871785270509090021, 0.008213979931070194626, 0.008556174591631299231, 0.008898369252192405571, 0.009240563912753511910, 0.009582758573314616515, 0.01026714789443683093, 0.01095153721555904534 ),
 .UNSPECIFIED. ) ;
#39866=( GEOMETRIC_REPRESENTATION_CONTEXT ( 3 ) GLOBAL_UNCERTAINTY_ASSIGNED_CONTEXT ( ( #55782 ) ) GLOBAL_UNIT_ASSIGNED_CONTEXT ( ( #14008, #238161, #139034 ) ) REPRESENTATION_CONTEXT ( 'NONE', 'WORKASPACE' ) );
#39938=DIRECTION ( 'NONE',  ( 0.8049926720990051576, 0.5932847527679298016, -0.000000000000000000 ) ) ;
#40128=VECTOR ( 'NONE', #192534, 1000.000000000000000 ) ;
#40144=DIRECTION ( 'NONE',  ( -0.000000000000000000, -0.000000000000000000, -1.000000000000000000 ) ) ;
#40377=EDGE_CURVE ( 'NONE', #816, #82768, #17460, .T. ) ;
#40603=FACE_OUTER_BOUND ( 'NONE', #109562, .T. ) ;
#40874=FACE_OUTER_BOUND ( 'NONE', #248392, .T. ) ;
#40903=EDGE_CURVE ( 'NONE', #222175, #101212, #78657, .T. ) ;
#41227=CARTESIAN_POINT ( 'NONE',  ( 21.72449340488910252, 10.28395627749111974, -9.250000000000001776 ) ) ;
#41692=DIRECTION ( 'NONE',  ( 1.186688945009010077E-16, -1.000000000000000000, -0.000000000000000000 ) ) ;
#41880=LINE ( 'NONE', #106948, #128634 ) ;
#41919=CARTESIAN_POINT ( 'NONE',  ( -14.45443560709636444, 9.450592112133699985, -15.05618831880839537 ) ) ;
#41951=VECTOR ( 'NONE', #67555, 1000.000000000000000 ) ;
#42235=ORIENTED_EDGE ( 'NONE', *, *, #179457, .T. ) ;
#42380=VERTEX_POINT ( 'NONE', #141009 ) ;
#42637=PLANE ( 'NONE',  #249614 ) ;
#42750=ORIENTED_EDGE ( 'NONE', *, *, #159260, .F. ) ;
#42788=CARTESIAN_POINT ( 'NONE',  ( -16.89318236219975944, 9.951535257875127272, -20.85512963210584658 ) ) ;
#42983=CARTESIAN_POINT ( 'NONE',  ( -14.45422546970484312, 9.450602096088523751, -18.44389596309667922 ) ) ;
#42989=EDGE_CURVE ( 'NONE', #17161, #254638, #190087, .T. ) ;
#43183=CARTESIAN_POINT ( 'NONE',  ( -13.54795643572458275, 9.450668889167525677, -15.05554649020735170 ) ) ;
#43202=CARTESIAN_POINT ( 'NONE',  ( -17.73285935861288110, 10.85798180379229372, -23.25856180978325938 ) ) ;
#43385=DIRECTION ( 'NONE',  ( -1.000000000000000000, 0.000000000000000000, 0.000000000000000000 ) ) ;
#43590=LINE ( 'NONE', #143958, #21199 ) ;
#43595=VECTOR ( 'NONE', #110496, 1000.000000000000000 ) ;
#43596=EDGE_LOOP ( 'NONE', ( #10978, #127204, #147980, #209517, #248039 ) ) ;
#43611=CARTESIAN_POINT ( 'NONE',  ( 14.88075390448863722, 9.431689550524096077, -18.27929003223605875 ) ) ;
#43613=CARTESIAN_POINT ( 'NONE',  ( -16.88783316861815109, 9.949999999999983302, -20.74773595802023962 ) ) ;
#43813=LINE ( 'NONE', #123352, #47740 ) ;
#43888=DIRECTION ( 'NONE',  ( -1.000000000000000000, 0.000000000000000000, 0.000000000000000000 ) ) ;
#43893=DIRECTION ( 'NONE',  ( 0.000000000000000000, 0.000000000000000000, 1.000000000000000000 ) ) ;
#43971=VERTEX_POINT ( 'NONE', #202309 ) ;
#44019=ORIENTED_EDGE ( 'NONE', *, *, #57281, .T. ) ;
#44132=( BOUNDED_SURFACE ( )  B_SPLINE_SURFACE ( 3, 2, ( 
 ( #48368, #243548, #104014 ),
 ( #221397, #226528, #62357 ),
 ( #63629, #67478, #246128 ),
 ( #42788, #162752, #4911 ) ),
 .UNSPECIFIED., .F., .F., .F. ) 
 B_SPLINE_SURFACE_WITH_KNOTS ( ( 4, 4 ),
 ( 3, 3 ),
 ( 0.0008258556059633722669, 0.0009616864997632808970 ),
 ( 0.000000000000000000, 1.000000000000000000 ),
 .UNSPECIFIED. ) 
 GEOMETRIC_REPRESENTATION_ITEM ( )  RATIONAL_B_SPLINE_SURFACE ( (
 ( 1.000000000000000000, 0.9152888060719368557, 1.000000000000000000),
 ( 1.000000000000000000, 0.9327727094138205111, 1.000000000000000000),
 ( 1.000000000000000000, 0.9369023509258461724, 1.000000000000000000),
 ( 1.000000000000000000, 0.9246339933864415883, 1.000000000000000000) ) ) 
 REPRESENTATION_ITEM ( '' )  SURFACE ( )  );
#44289=CARTESIAN_POINT ( 'NONE',  ( -17.04761207306817994, 10.02645087339777064, -20.85000000000000142 ) ) ;
#44478=EDGE_CURVE ( 'NONE', #199540, #64185, #171567, .T. ) ;
#44779=DIRECTION ( 'NONE',  ( 0.7071067811865487940, 0.7071067811865462405, -7.215498431451186046E-16 ) ) ;
#44903=CARTESIAN_POINT ( 'NONE',  ( -16.83794479845801817, 9.926357419351495182, -20.69644470422230853 ) ) ;
#45065=VERTEX_POINT ( 'NONE', #120285 ) ;
#45171=CARTESIAN_POINT ( 'NONE',  ( 16.27683809663750125, 9.349999999999983658, -9.250000000000001776 ) ) ;
#45198=LINE ( 'NONE', #4760, #145457 ) ;
#45294=AXIS2_PLACEMENT_3D ( 'NONE', #240340, #179106, #162093 ) ;
#45343=DIRECTION ( 'NONE',  ( -1.000000000000000000, 0.000000000000000000, 0.000000000000000000 ) ) ;
#45441=ORIENTED_EDGE ( 'NONE', *, *, #151832, .T. ) ;
#45508=EDGE_CURVE ( 'NONE', #54287, #214183, #208339, .T. ) ;
#45519=CARTESIAN_POINT ( 'NONE',  ( -18.40000000000000213, 11.74999999999998224, -24.25000000000001066 ) ) ;
#45525=FACE_OUTER_BOUND ( 'NONE', #99402, .T. ) ;
#45739=CARTESIAN_POINT ( 'NONE',  ( -15.39946565075089779, 9.389534562346700142, -15.67480930438995479 ) ) ;
#45879=CARTESIAN_POINT ( 'NONE',  ( 18.54999999999999716, 8.750000000000024869, -20.85000000000000142 ) ) ;
#45994=ORIENTED_EDGE ( 'NONE', *, *, #127616, .T. ) ;
#46103=EDGE_CURVE ( 'NONE', #12920, #194069, #181192, .T. ) ;
#46172=DIRECTION ( 'NONE',  ( -1.000000000000000000, -1.646408749285562691E-14, 0.000000000000000000 ) ) ;
#46266=CARTESIAN_POINT ( 'NONE',  ( -16.80117486205003630, 9.949657268312314784, -20.84885487292548589 ) ) ;
#46336=B_SPLINE_CURVE_WITH_KNOTS ( 'NONE', 3,
 ( #13689, #194922, #252287, #254816, #54097, #236577, #134894, #74982, #215728, #76219, #232760, #116645, #253575, #196184, #133640, #154529, #17529, #97034, #57936, #234018, #137473, #217014, #34561, #38396, #197458, #18823 ),
 .UNSPECIFIED., .F., .F.,
 ( 4, 2, 2, 2, 2, 2, 2, 2, 2, 2, 2, 2, 4 ),
 ( 0.005476422646581347378, 0.006160811967703559190, 0.006845201288825771002, 0.007187395949386877342, 0.007529590609947982814, 0.007871785270509088286, 0.008213979931070194626, 0.008556174591631300966, 0.008898369252192407305, 0.009240563912753511910, 0.009582758573314618250, 0.01026714789443682746, 0.01095153721555903494 ),
 .UNSPECIFIED. ) ;
#46443=DIRECTION ( 'NONE',  ( 1.186688945009009831E-16, -1.000000000000000000, 0.000000000000000000 ) ) ;
#46608=DIRECTION ( 'NONE',  ( -1.073024830501117725E-15, 0.000000000000000000, -1.000000000000000000 ) ) ;
#46631=ORIENTED_EDGE ( 'NONE', *, *, #233760, .F. ) ;
#46646=AXIS2_PLACEMENT_3D ( 'NONE', #165124, #60876, #103840 ) ;
#46716=ADVANCED_FACE ( 'NONE', ( #13778 ), #148148, .F. ) ;
#46784=LINE ( 'NONE', #45519, #120279 ) ;
#46994=ORIENTED_EDGE ( 'NONE', *, *, #235919, .F. ) ;
#47194=AXIS2_PLACEMENT_3D ( 'NONE', #255955, #117782, #76085 ) ;
#47299=( NAMED_UNIT ( * ) PLANE_ANGLE_UNIT ( ) SI_UNIT ( $, .RADIAN. ) );
#47344=VERTEX_POINT ( 'NONE', #45879 ) ;
#47543=CARTESIAN_POINT ( 'NONE',  ( -16.77683809663752257, 9.945835743204147761, -20.83605098089580210 ) ) ;
#47629=CARTESIAN_POINT ( 'NONE',  ( -16.94107738177414291, 10.01423928513661998, -20.94999999999999929 ) ) ;
#47717=DIRECTION ( 'NONE',  ( 0.5932847527679310229, -0.8049926720990042694, -6.366092712777067056E-16 ) ) ;
#47740=VECTOR ( 'NONE', #184595, 1000.000000000000000 ) ;
#47766=VERTEX_POINT ( 'NONE', #68661 ) ;
#47838=EDGE_LOOP ( 'NONE', ( #48013, #35378, #104169, #246196, #127521, #32855, #134166, #150997, #179287, #29270, #239853, #59913, #243314, #129255 ) ) ;
#47856=CARTESIAN_POINT ( 'NONE',  ( -16.87851181299898684, 9.950042924007739487, -12.64985648463308365 ) ) ;
#47941=CARTESIAN_POINT ( 'NONE',  ( -23.25000000000000355, 11.74999999999998224, -9.250000000000001776 ) ) ;
#47942=CARTESIAN_POINT ( 'NONE',  ( -18.40000000000000213, 11.74999999999998224, -20.85000000000000142 ) ) ;
#48013=ORIENTED_EDGE ( 'NONE', *, *, #122043, .F. ) ;
#48122=CARTESIAN_POINT ( 'NONE',  ( 20.27550659511088682, 9.216043722508844738, -9.250000000000001776 ) ) ;
#48155=DIRECTION ( 'NONE',  ( 0.000000000000000000, -1.000000000000000000, 0.000000000000000000 ) ) ;
#48197=CARTESIAN_POINT ( 'NONE',  ( -21.65000000000000213, 7.249999999999983125, -9.250000000000001776 ) ) ;
#48208=EDGE_CURVE ( 'NONE', #166202, #42380, #52631, .T. ) ;
#48368=CARTESIAN_POINT ( 'NONE',  ( -16.87036670365548474, 9.989418819301645769, -20.97956011730205006 ) ) ;
#48592=ORIENTED_EDGE ( 'NONE', *, *, #40377, .T. ) ;
#48681=CARTESIAN_POINT ( 'NONE',  ( -21.65000000000000213, 9.949999999999983302, -12.75000000000000178 ) ) ;
#48840=CARTESIAN_POINT ( 'NONE',  ( -18.40000000000000213, 11.41458325959978382, -12.65000000000000213 ) ) ;
#49040=CARTESIAN_POINT ( 'NONE',  ( -16.94333152886235894, 9.990342011450481507, -12.60796846894558954 ) ) ;
#49058=AXIS2_PLACEMENT_3D ( 'NONE', #140060, #114091, #193649 ) ;
#49159=CARTESIAN_POINT ( 'NONE',  ( -20.65000000000000568, 7.249999999999983125, -20.85000000000000142 ) ) ;
#49281=DIRECTION ( 'NONE',  ( -0.000000000000000000, 1.000000000000000000, -0.000000000000000000 ) ) ;
#49327=CIRCLE ( 'NONE', #195093, 14.30833333333333890 ) ;
#49360=EDGE_CURVE ( 'NONE', #196735, #27978, #49327, .T. ) ;
#49380=CARTESIAN_POINT ( 'NONE',  ( 20.27550659511089037, 9.216043722508848290, -12.65000000000000391 ) ) ;
#49475=CARTESIAN_POINT ( 'NONE',  ( -18.39999999999999858, 11.47316190336247388, -9.325946066807970780 ) ) ;
#49489=DIRECTION ( 'NONE',  ( 0.000000000000000000, 0.000000000000000000, 1.000000000000000000 ) ) ;
#49644=ORIENTED_EDGE ( 'NONE', *, *, #22727, .F. ) ;
#49751=EDGE_CURVE ( 'NONE', #208072, #116233, #155232, .T. ) ;
#49948=CARTESIAN_POINT ( 'NONE',  ( -17.01764560440441088, 9.949999999999983302, -20.75000000078611251 ) ) ;
#50176=ADVANCED_FACE ( 'NONE', ( #120924 ), #42637, .F. ) ;
#50218=ORIENTED_EDGE ( 'NONE', *, *, #200022, .T. ) ;
#50443=DIRECTION ( 'NONE',  ( 1.186688945009010077E-16, -1.000000000000000000, -0.000000000000000000 ) ) ;
#50518=ORIENTED_EDGE ( 'NONE', *, *, #128569, .F. ) ;
#50661=CARTESIAN_POINT ( 'NONE',  ( -17.71734398241073905, 10.84235722846456085, -10.27486174699440724 ) ) ;
#50885=VERTEX_POINT ( 'NONE', #220357 ) ;
#50933=VECTOR ( 'NONE', #13843, 1000.000000000000000 ) ;
#51112=VERTEX_POINT ( 'NONE', #91101 ) ;
#51271=CARTESIAN_POINT ( 'NONE',  ( -16.83558968593870731, 9.949999999999983302, -12.66230518761681445 ) ) ;
#51288=CARTESIAN_POINT ( 'NONE',  ( -18.34374000495059676, 11.47316190336247388, -24.25000000000001066 ) ) ;
#51315=EDGE_CURVE ( 'NONE', #212402, #217199, #257817, .T. ) ;
#51555=VECTOR ( 'NONE', #38219, 1000.000000000000000 ) ;
#51569=DIRECTION ( 'NONE',  ( 0.7071067811865463515, -0.7071067811865487940, 4.930380657631324879E-32 ) ) ;
#51793=DIRECTION ( 'NONE',  ( 0.2834754621636358940, -0.2834754621636437211, 0.9161240771326893961 ) ) ;
#51880=EDGE_CURVE ( 'NONE', #106685, #109071, #99553, .T. ) ;
#51881=VECTOR ( 'NONE', #234286, 1000.000000000000000 ) ;
#51944=CARTESIAN_POINT ( 'NONE',  ( -18.34374000495060386, 11.47316190336247033, -9.249999999999998224 ) ) ;
#52068=ORIENTED_EDGE ( 'NONE', *, *, #51880, .F. ) ;
#52201=ORIENTED_EDGE ( 'NONE', *, *, #39456, .T. ) ;
#52295=MECHANICAL_DESIGN_GEOMETRIC_PRESENTATION_REPRESENTATION('',(#89720),#39866);
#52443=DIRECTION ( 'NONE',  ( -1.000000000000000000, 0.000000000000000000, 0.000000000000000000 ) ) ;
#52578=CARTESIAN_POINT ( 'NONE',  ( -16.87683809663750267, 9.949999999999983302, -13.40236401819648115 ) ) ;
#52631=LINE ( 'NONE', #187043, #185262 ) ;
#53310=LINE ( 'NONE', #14206, #240439 ) ;
#53539=VERTEX_POINT ( 'NONE', #100236 ) ;
#53645=ORIENTED_EDGE ( 'NONE', *, *, #99249, .F. ) ;
#53666=ADVANCED_FACE ( 'NONE', ( #211557 ), #15952, .F. ) ;
#53880=CARTESIAN_POINT ( 'NONE',  ( -16.89155683852557743, 9.949999999999981526, -13.27737184954015603 ) ) ;
#53933=CARTESIAN_POINT ( 'NONE',  ( -16.97048361161166952, 9.949999999999981526, -20.35888434443039685 ) ) ;
#53981=DIRECTION ( 'NONE',  ( -0.7071067811865487940, 0.7071067811865463515, -7.215498431451184074E-16 ) ) ;
#53993=DIRECTION ( 'NONE',  ( 1.000000000000000000, 0.000000000000000000, 0.000000000000000000 ) ) ;
#54097=CARTESIAN_POINT ( 'NONE',  ( 12.60053434924910576, 9.389534562346701918, -15.67480930438995479 ) ) ;
#54169=ADVANCED_FACE ( 'NONE', ( #128510 ), #28151, .F. ) ;
#54183=ADVANCED_FACE ( 'NONE', ( #12434 ), #192336, .F. ) ;
#54287=VERTEX_POINT ( 'NONE', #172814 ) ;
#54298=DIRECTION ( 'NONE',  ( 0.000000000000000000, 0.000000000000000000, 1.000000000000000000 ) ) ;
#54401=SHAPE_REPRESENTATION_RELATIONSHIP ( 'NONE' , 'NONE' ,  #224939, #144531 ) ;
#54545=DIRECTION ( 'NONE',  ( 1.000000000000000000, 0.000000000000000000, 0.000000000000000000 ) ) ;
#54902=ORIENTED_EDGE ( 'NONE', *, *, #89182, .F. ) ;
#55123=CARTESIAN_POINT ( 'NONE',  ( -16.96982749440708815, 9.949999999999983302, -13.12477840881186530 ) ) ;
#55176=CARTESIAN_POINT ( 'NONE',  ( -16.84419801905645286, 9.949999999999985079, -20.83051015377798265 ) ) ;
#55242=DIRECTION ( 'NONE',  ( 1.000000000000000000, 0.000000000000000000, -0.000000000000000000 ) ) ;
#55278=CARTESIAN_POINT ( 'NONE',  ( -16.87036670365549895, 9.989418819301647545, -12.52043988269794639 ) ) ;
#55522=CARTESIAN_POINT ( 'NONE',  ( 16.87683809663750267, 9.949999999999983302, -12.65000000000000036 ) ) ;
#55782=UNCERTAINTY_MEASURE_WITH_UNIT (LENGTH_MEASURE( 1.000000000000000082E-05 ), #14008, 'distance_accuracy_value', 'NONE');
#56073=CARTESIAN_POINT ( 'NONE',  ( 18.39999999999999503, 11.74999999999998224, -12.65000000000000213 ) ) ;
#56112=CARTESIAN_POINT ( 'NONE',  ( -16.81744102076749314, 9.949999999999986855, -12.65000000000000213 ) ) ;
#56132=ORIENTED_EDGE ( 'NONE', *, *, #139542, .T. ) ;
#56289=VECTOR ( 'NONE', #77333, 999.9999999999998863 ) ;
#56522=CARTESIAN_POINT ( 'NONE',  ( 16.27683809663749770, 9.349999999999983658, -9.250000000000005329 ) ) ;
#56757=CARTESIAN_POINT ( 'NONE',  ( 18.54999999999999716, 8.750000000000024869, -9.250000000000001776 ) ) ;
#56794=LINE ( 'NONE', #18974, #72648 ) ;
#57030=DIRECTION ( 'NONE',  ( -0.000000000000000000, 1.000000000000000000, -0.000000000000000000 ) ) ;
#57067=ORIENTED_EDGE ( 'NONE', *, *, #85243, .T. ) ;
#57144=CARTESIAN_POINT ( 'NONE',  ( -16.91049119928364419, 9.949999999999983302, -12.61827960680916405 ) ) ;
#57281=EDGE_CURVE ( 'NONE', #83518, #92740, #22621, .T. ) ;
#57436=DIRECTION ( 'NONE',  ( 0.000000000000000000, 0.000000000000000000, -1.000000000000000000 ) ) ;
#57495=ORIENTED_EDGE ( 'NONE', *, *, #42989, .T. ) ;
#57717=ORIENTED_EDGE ( 'NONE', *, *, #51315, .T. ) ;
#57768=( BOUNDED_CURVE ( )  B_SPLINE_CURVE ( 3, ( #193086, #93963, #195667, #131811 ),
 .UNSPECIFIED., .F., .F. ) 
 B_SPLINE_CURVE_WITH_KNOTS ( ( 4, 4 ),
 ( 0.5235987755983007030, 1.570796326794896558 ),
 .UNSPECIFIED. ) 
 CURVE ( )  GEOMETRIC_REPRESENTATION_ITEM ( )  RATIONAL_B_SPLINE_CURVE ( ( 1.000000000000000000, 0.9106836025229594345, 0.9106836025229594345, 1.000000000000000000 ) ) 
 REPRESENTATION_ITEM ( '' )  );
#57883=CARTESIAN_POINT ( 'NONE',  ( -16.88005004766534967, 9.950100503321044343, -20.85033611194876002 ) ) ;
#57936=CARTESIAN_POINT ( 'NONE',  ( 14.87567385445977486, 9.430764995422318719, -15.23053739475045809 ) ) ;
#57982=CARTESIAN_POINT ( 'NONE',  ( -18.40000000000000213, 11.47316190336247388, -12.55000000000000249 ) ) ;
#58005=CARTESIAN_POINT ( 'NONE',  ( -16.79814274880124358, 9.949272542677302766, -12.65243303704799693 ) ) ;
#58080=EDGE_LOOP ( 'NONE', ( #211951, #119044, #212154, #157284, #183470, #81090, #193201, #190199, #132479, #137600 ) ) ;
#58165=DIRECTION ( 'NONE',  ( -0.5932847527679298016, 0.8049926720990051576, 0.000000000000000000 ) ) ;
#58471=CARTESIAN_POINT ( 'NONE',  ( -18.34374000495060386, 11.47316190336247033, -9.249999999999998224 ) ) ;
#58499=ORIENTED_EDGE ( 'NONE', *, *, #106316, .T. ) ;
#58573=ORIENTED_EDGE ( 'NONE', *, *, #191285, .T. ) ;
#58709=CARTESIAN_POINT ( 'NONE',  ( -17.78241384943093095, 10.85557575278284226, -10.24903767247034914 ) ) ;
#58913=ORIENTED_EDGE ( 'NONE', *, *, #87942, .T. ) ;
#58924=CARTESIAN_POINT ( 'NONE',  ( -16.94052228080551714, 9.986279733098838207, -20.89037550266942134 ) ) ;
#58955=DIRECTION ( 'NONE',  ( -1.073024830501117725E-15, 0.000000000000000000, 1.000000000000000000 ) ) ;
#58965=DIRECTION ( 'NONE',  ( -0.000000000000000000, -0.000000000000000000, -1.000000000000000000 ) ) ;
#59104=FACE_OUTER_BOUND ( 'NONE', #193306, .T. ) ;
#59150=CARTESIAN_POINT ( 'NONE',  ( -16.89146115310546037, 9.951443245656456327, -20.85482241895421751 ) ) ;
#59181=ORIENTED_EDGE ( 'NONE', *, *, #236971, .T. ) ;
#59268=CARTESIAN_POINT ( 'NONE',  ( -16.97683809663752186, 9.949999999999983302, -20.09763598180368405 ) ) ;
#59676=ORIENTED_EDGE ( 'NONE', *, *, #247500, .F. ) ;
#59828=VECTOR ( 'NONE', #13218, 1000.000000000000000 ) ;
#59913=ORIENTED_EDGE ( 'NONE', *, *, #179288, .F. ) ;
#60528=EDGE_LOOP ( 'NONE', ( #21286, #176872, #157680, #58913 ) ) ;
#60537=ORIENTED_EDGE ( 'NONE', *, *, #102853, .T. ) ;
#60583=CARTESIAN_POINT ( 'NONE',  ( -16.78569801330231925, 9.947933733113496046, -12.65691290534750024 ) ) ;
#60760=VERTEX_POINT ( 'NONE', #240544 ) ;
#60876=DIRECTION ( 'NONE',  ( 1.186688945009010077E-16, -1.000000000000000000, -0.000000000000000000 ) ) ;
#61302=ORIENTED_EDGE ( 'NONE', *, *, #81866, .T. ) ;
#61397=VECTOR ( 'NONE', #68176, 1000.000000000000000 ) ;
#61421=PRODUCT_DEFINITION_FORMATION_WITH_SPECIFIED_SOURCE ( 'ANY', '', #149326, .NOT_KNOWN. ) ;
#61479=FACE_OUTER_BOUND ( 'NONE', #239974, .T. ) ;
#61746=VECTOR ( 'NONE', #25834, 1000.000000000000000 ) ;
#61758=LINE ( 'NONE', #220826, #16369 ) ;
#61888=CARTESIAN_POINT ( 'NONE',  ( -16.81744102076749314, 9.949999999999986855, -12.65000000000000213 ) ) ;
#61916=CARTESIAN_POINT ( 'NONE',  ( -18.39418127959864790, 11.48390560169813668, -24.25000000000000000 ) ) ;
#62346=DIRECTION ( 'NONE',  ( -1.000000000000000000, 0.000000000000000000, 0.000000000000000000 ) ) ;
#62348=CIRCLE ( 'NONE', #221110, 0.09999999999999939493 ) ;
#62357=CARTESIAN_POINT ( 'NONE',  ( -16.92778301347278358, 10.00094491683526066, -20.92851810796845413 ) ) ;
#62744=CARTESIAN_POINT ( 'NONE',  ( -12.25000000000000178, 9.349999999999980105, -16.51856895740264264 ) ) ;
#63160=CARTESIAN_POINT ( 'NONE',  ( -16.81931177881022776, 9.936996059503902856, -20.77321787861722413 ) ) ;
#63181=CARTESIAN_POINT ( 'NONE',  ( -18.34374000495059676, 11.47316190336247388, -24.25000000000001066 ) ) ;
#63409=CARTESIAN_POINT ( 'NONE',  ( -16.90202395485773224, 9.965944544550314532, -12.59698627874055354 ) ) ;
#63580=CARTESIAN_POINT ( 'NONE',  ( -16.88560720703333473, 9.950564843749692301, -12.64811192086371783 ) ) ;
#63622=CARTESIAN_POINT ( 'NONE',  ( 20.04999999999999716, 8.750000000000014211, -9.250000000000001776 ) ) ;
#63629=CARTESIAN_POINT ( 'NONE',  ( -16.86445178670652467, 9.962211629115985900, -20.89077743811727572 ) ) ;
#63705=DIRECTION ( 'NONE',  ( 0.000000000000000000, 0.000000000000000000, -1.000000000000000000 ) ) ;
#64023=CARTESIAN_POINT ( 'NONE',  ( -13.88555196119803625, 9.457431528848909252, -14.99991693789966085 ) ) ;
#64185=VERTEX_POINT ( 'NONE', #89614 ) ;
#64703=CARTESIAN_POINT ( 'NONE',  ( -16.94107738177415712, 10.01423928513661821, -12.55000000000000249 ) ) ;
#64852=FACE_OUTER_BOUND ( 'NONE', #168583, .T. ) ;
#64947=ORIENTED_EDGE ( 'NONE', *, *, #67308, .F. ) ;
#65260=CARTESIAN_POINT ( 'NONE',  ( 16.87683809663750267, 9.949999999999983302, -12.65000000000000036 ) ) ;
#65492=CARTESIAN_POINT ( 'NONE',  ( 18.39999999999999503, 11.47316190336248454, -24.25000000000001066 ) ) ;
#65722=ORIENTED_EDGE ( 'NONE', *, *, #101380, .F. ) ;
#65736=CARTESIAN_POINT ( 'NONE',  ( -16.80891096016321384, 9.949999999999983302, -20.86766280726859080 ) ) ;
#65914=PRODUCT_DEFINITION_SHAPE ( 'NONE', 'NONE',  #97863 ) ;
#66368=CARTESIAN_POINT ( 'NONE',  ( -16.93909480342659890, 9.993078364801540658, -12.60034701667233037 ) ) ;
#66820=DIRECTION ( 'NONE',  ( -0.000000000000000000, -0.000000000000000000, -1.000000000000000000 ) ) ;
#66958=ADVANCED_FACE ( 'NONE', ( #196205 ), #136197, .F. ) ;
#67022=CARTESIAN_POINT ( 'NONE',  ( 15.74999999999999645, 9.349999999999983658, -16.75000000000000000 ) ) ;
#67128=CARTESIAN_POINT ( 'NONE',  ( -16.78270389226382875, 9.947372616617009555, -20.84120703691148080 ) ) ;
#67308=EDGE_CURVE ( 'NONE', #92740, #88402, #235947, .T. ) ;
#67478=CARTESIAN_POINT ( 'NONE',  ( -16.90202395485793829, 9.965944544550675133, -20.90301372125983193 ) ) ;
#67547=EDGE_CURVE ( 'NONE', #106852, #27978, #247928, .T. ) ;
#67555=DIRECTION ( 'NONE',  ( 1.000000000000000000, -0.000000000000000000, -0.000000000000000000 ) ) ;
#67559=CARTESIAN_POINT ( 'NONE',  ( -16.87304349924914604, 9.961745077957175454, -20.88906667504524961 ) ) ;
#67621=ADVANCED_FACE ( 'NONE', ( #248238 ), #246938, .F. ) ;
#67632=LINE ( 'NONE', #166771, #117007 ) ;
#67668=CARTESIAN_POINT ( 'NONE',  ( -15.31895204843005587, 9.396533993953919861, -17.90593977917330193 ) ) ;
#67755=CARTESIAN_POINT ( 'NONE',  ( -18.39999999999999858, 11.47316190336247388, -9.299829248466007670 ) ) ;
#67836=VERTEX_POINT ( 'NONE', #130851 ) ;
#67881=DIRECTION ( 'NONE',  ( -0.000000000000000000, -0.000000000000000000, -1.000000000000000000 ) ) ;
#68028=DIRECTION ( 'NONE',  ( -0.7071067811865456854, 0.7071067811865493491, 0.000000000000000000 ) ) ;
#68176=DIRECTION ( 'NONE',  ( -0.000000000000000000, -0.000000000000000000, -1.000000000000000000 ) ) ;
#68206=DIRECTION ( 'NONE',  ( 1.000000000000000000, 0.000000000000000000, 1.073024830501117725E-15 ) ) ;
#68322=DIRECTION ( 'NONE',  ( -1.646408749285562691E-14, 1.000000000000000000, 0.000000000000000000 ) ) ;
#68437=VERTEX_POINT ( 'NONE', #102957 ) ;
#68478=ORIENTED_EDGE ( 'NONE', *, *, #78632, .F. ) ;
#68661=CARTESIAN_POINT ( 'NONE',  ( -16.87331047859651179, 9.949999999999986855, -12.65000000000000213 ) ) ;
#68983=ORIENTED_EDGE ( 'NONE', *, *, #202132, .F. ) ;
#69418=CARTESIAN_POINT ( 'NONE',  ( 21.72449340488910607, 10.28395627749111441, -20.84999999999999787 ) ) ;
#69473=DIRECTION ( 'NONE',  ( -1.000000000000000000, 3.854941057726231589E-15, 1.927470528863115795E-15 ) ) ;
#69540=CARTESIAN_POINT ( 'NONE',  ( -16.92209698673574181, 9.949999999999983302, -20.78936443294790237 ) ) ;
#69603=CARTESIAN_POINT ( 'NONE',  ( -16.87998658237743754, 9.949999999999985079, -12.86363956773800510 ) ) ;
#69674=VECTOR ( 'NONE', #1447, 1000.000000000000000 ) ;
#69940=ORIENTED_EDGE ( 'NONE', *, *, #179457, .F. ) ;
#70024=AXIS2_PLACEMENT_3D ( 'NONE', #47941, #170527, #173088 ) ;
#70034=ADVANCED_FACE ( 'NONE', ( #64852 ), #28343, .F. ) ;
#70773=EDGE_CURVE ( 'NONE', #118880, #194069, #245473, .T. ) ;
#70901=CARTESIAN_POINT ( 'NONE',  ( -16.93710578446424009, 9.949999999999983302, -12.91880398379939265 ) ) ;
#70907=CARTESIAN_POINT ( 'NONE',  ( -16.83558968593875349, 9.949999999999983302, -20.83769481238317667 ) ) ;
#71101=VERTEX_POINT ( 'NONE', #142052 ) ;
#71137=DIRECTION ( 'NONE',  ( -1.000000000000000000, 0.000000000000000000, 0.000000000000000000 ) ) ;
#71191=LINE ( 'NONE', #248522, #213473 ) ;
#71231=ORIENTED_EDGE ( 'NONE', *, *, #89002, .T. ) ;
#71251=EDGE_CURVE ( 'NONE', #248097, #217199, #167859, .T. ) ;
#71525=EDGE_CURVE ( 'NONE', #75919, #196737, #183238, .T. ) ;
#71527=CARTESIAN_POINT ( 'NONE',  ( -16.94107738177415712, 10.01423928513662176, -12.55000000000000249 ) ) ;
#71892=EDGE_CURVE ( 'NONE', #54287, #7235, #242899, .T. ) ;
#71917=DIRECTION ( 'NONE',  ( 1.000000000000000000, 0.000000000000000000, 0.000000000000000000 ) ) ;
#72160=ORIENTED_EDGE ( 'NONE', *, *, #226076, .T. ) ;
#72648=VECTOR ( 'NONE', #195084, 1000.000000000000000 ) ;
#72714=ORIENTED_EDGE ( 'NONE', *, *, #17399, .T. ) ;
#72906=EDGE_LOOP ( 'NONE', ( #20521, #144534, #126974 ) ) ;
#72913=EDGE_CURVE ( 'NONE', #118880, #125620, #214390, .T. ) ;
#73328=CARTESIAN_POINT ( 'NONE',  ( -17.11825945287481332, 9.949999999999983302, -20.75000000000000000 ) ) ;
#73432=DIRECTION ( 'NONE',  ( 1.000000000000000000, 0.000000000000000000, 0.000000000000000000 ) ) ;
#73782=CARTESIAN_POINT ( 'NONE',  ( 20.73486653747088937, 7.750000000000025757, -12.65000000000000568 ) ) ;
#73798=AXIS2_PLACEMENT_3D ( 'NONE', #41227, #39938, #58165 ) ;
#73843=AXIS2_PLACEMENT_3D ( 'NONE', #149157, #68322, #46172 ) ;
#73895=ORIENTED_EDGE ( 'NONE', *, *, #229633, .T. ) ;
#74010=SURFACE_SIDE_STYLE ('',( #257675 ) ) ;
#74141=CARTESIAN_POINT ( 'NONE',  ( -16.80468759584938709, 9.942153675134134616, -12.69001886620163688 ) ) ;
#74764=CARTESIAN_POINT ( 'NONE',  ( -16.87683809663752754, 9.865889849332413419, -13.26742680706974831 ) ) ;
#74784=CARTESIAN_POINT ( 'NONE',  ( -16.77683809663752257, 9.945835743204145984, -12.66394901910421034 ) ) ;
#74830=DIRECTION ( 'NONE',  ( 1.000000000000000000, 0.000000000000000000, 0.000000000000000000 ) ) ;
#74881=CARTESIAN_POINT ( 'NONE',  ( -18.39999999999999858, 11.47316190336247388, -9.325946066807970780 ) ) ;
#74982=CARTESIAN_POINT ( 'NONE',  ( 13.12220780326571834, 9.430633469072795094, -15.23176579482408322 ) ) ;
#75103=ORIENTED_EDGE ( 'NONE', *, *, #251969, .T. ) ;
#75900=DIRECTION ( 'NONE',  ( -0.000000000000000000, -0.000000000000000000, -1.000000000000000000 ) ) ;
#75919=VERTEX_POINT ( 'NONE', #217833 ) ;
#75959=CARTESIAN_POINT ( 'NONE',  ( -16.92563707711778420, 9.968990694396778096, -20.88075829952397555 ) ) ;
#76085=DIRECTION ( 'NONE',  ( 0.000000000000000000, 0.000000000000000000, 1.000000000000000000 ) ) ;
#76165=LINE ( 'NONE', #158323, #119675 ) ;
#76219=CARTESIAN_POINT ( 'NONE',  ( 13.43443725621852458, 9.446557523072529605, -15.08994195434588370 ) ) ;
#76293=CARTESIAN_POINT ( 'NONE',  ( -16.77977881697927032, 9.946601933532905448, -12.66137857311505499 ) ) ;
#76450=EDGE_CURVE ( 'NONE', #75919, #223695, #114283, .T. ) ;
#77008=CARTESIAN_POINT ( 'NONE',  ( -17.27223548803747377, 10.34539739140543269, -11.36639382080207028 ) ) ;
#77264=ORIENTED_EDGE ( 'NONE', *, *, #116110, .F. ) ;
#77333=DIRECTION ( 'NONE',  ( -0.7071067811865463515, -0.7071067811865487940, 7.587431340288849180E-16 ) ) ;
#77645=ORIENTED_EDGE ( 'NONE', *, *, #227411, .T. ) ;
#78253=CARTESIAN_POINT ( 'NONE',  ( -16.97683809663752896, 9.949999999999986855, -13.27152476866994490 ) ) ;
#78283=CARTESIAN_POINT ( 'NONE',  ( -18.37013991200266005, 11.49974761621196961, -9.206976989482884122 ) ) ;
#78506=CARTESIAN_POINT ( 'NONE',  ( -16.93935632781549572, 9.984730499725088748, -20.88966074871030187 ) ) ;
#78622=ORIENTED_EDGE ( 'NONE', *, *, #236403, .T. ) ;
#78632=EDGE_CURVE ( 'NONE', #7235, #249899, #164427, .T. ) ;
#78657=CIRCLE ( 'NONE', #107712, 1.749999999999998002 ) ;
#78893=AXIS2_PLACEMENT_3D ( 'NONE', #7551, #51793, #171799 ) ;
#78925=B_SPLINE_CURVE_WITH_KNOTS ( 'NONE', 3,
 ( #157028, #236530, #57883, #216961, #38353, #117870, #197408, #59150, #5607, #86423 ),
 .UNSPECIFIED., .F., .F.,
 ( 4, 3, 3, 4 ),
 ( 0.000000000000000000, 1.004626015991467516E-05, 1.831183478183015626E-05, 2.062343583996046153E-05 ),
 .UNSPECIFIED. ) ;
#79075=PRESENTATION_STYLE_ASSIGNMENT (( #195232 ) ) ;
#79156=CARTESIAN_POINT ( 'NONE',  ( -18.39999999999999858, 11.41458325959979625, -20.85000000000000142 ) ) ;
#79249=EDGE_CURVE ( 'NONE', #140980, #219433, #46336, .T. ) ;
#79865=CARTESIAN_POINT ( 'NONE',  ( 18.54999999999999716, 8.750000000000024869, -20.85000000000000142 ) ) ;
#80182=DIRECTION ( 'NONE',  ( -1.000000000000000000, -0.000000000000000000, -0.000000000000000000 ) ) ;
#80320=CARTESIAN_POINT ( 'NONE',  ( -18.40000000000000213, 5.649999999999983480, -12.65000000000000213 ) ) ;
#80602=AXIS2_PLACEMENT_3D ( 'NONE', #168486, #169759, #71917 ) ;
#80790=CARTESIAN_POINT ( 'NONE',  ( -13.77083647240106323, 9.457410930290160778, -18.49991590874628855 ) ) ;
#80830=FACE_OUTER_BOUND ( 'NONE', #12996, .T. ) ;
#81090=ORIENTED_EDGE ( 'NONE', *, *, #229317, .T. ) ;
#81209=ORIENTED_EDGE ( 'NONE', *, *, #167727, .T. ) ;
#81235=ORIENTED_EDGE ( 'NONE', *, *, #44478, .T. ) ;
#81694=( BOUNDED_CURVE ( )  B_SPLINE_CURVE ( 3, ( #166356, #224981, #26839, #47629 ),
 .UNSPECIFIED., .F., .T. ) 
 B_SPLINE_CURVE_WITH_KNOTS ( ( 4, 4 ),
 ( 5.733388419619901200, 5.983100554402347449 ),
 .UNSPECIFIED. ) 
 CURVE ( )  GEOMETRIC_REPRESENTATION_ITEM ( )  RATIONAL_B_SPLINE_CURVE ( ( 1.000000000000000000, 0.9948104011409417691, 0.9948104011409417691, 1.000000000000000000 ) ) 
 REPRESENTATION_ITEM ( '' )  );
#81714=EDGE_CURVE ( 'NONE', #200257, #194069, #45198, .T. ) ;
#81849=ORIENTED_EDGE ( 'NONE', *, *, #180090, .F. ) ;
#81866=EDGE_CURVE ( 'NONE', #64185, #54287, #149782, .T. ) ;
#82033=CARTESIAN_POINT ( 'NONE',  ( 23.24999999999999645, 5.649999999999983480, -20.84999999999999432 ) ) ;
#82282=EDGE_LOOP ( 'NONE', ( #164243, #176885, #151210, #52068 ) ) ;
#82661=DIRECTION ( 'NONE',  ( -1.000000000000000000, 0.000000000000000000, 1.156482317317870344E-15 ) ) ;
#82712=ORIENTED_EDGE ( 'NONE', *, *, #106316, .F. ) ;
#82768=VERTEX_POINT ( 'NONE', #39184 ) ;
#82901=EDGE_LOOP ( 'NONE', ( #102999, #210561, #228344, #183229 ) ) ;
#82951=CARTESIAN_POINT ( 'NONE',  ( -16.97683809663752186, 9.949999999999983302, -20.09763598180368405 ) ) ;
#82978=LINE ( 'NONE', #105106, #4939 ) ;
#83123=EDGE_CURVE ( 'NONE', #53539, #201670, #200163, .T. ) ;
#83518=VERTEX_POINT ( 'NONE', #117748 ) ;
#83552=CARTESIAN_POINT ( 'NONE',  ( -12.60206096961792532, 9.389686005655656587, -15.67284350635130430 ) ) ;
#83864=CARTESIAN_POINT ( 'NONE',  ( 18.39999999999999503, 5.649999999999983480, -20.85000000000000142 ) ) ;
#83962=CARTESIAN_POINT ( 'NONE',  ( 13.88638282980483574, 9.457426452488901347, -18.50004186840002873 ) ) ;
#83963=CARTESIAN_POINT ( 'NONE',  ( -16.93710578446422943, 9.949999999999983302, -20.58119601620066064 ) ) ;
#84028=AXIS2_PLACEMENT_3D ( 'NONE', #45171, #21775, #43893 ) ;
#84176=ORIENTED_EDGE ( 'NONE', *, *, #105804, .T. ) ;
#84240=PLANE ( 'NONE',  #84028 ) ;
#84260=CARTESIAN_POINT ( 'NONE',  ( -16.94275863009466576, 9.989496048662386940, -12.60830261795888241 ) ) ;
#84476=AXIS2_PLACEMENT_3D ( 'NONE', #257145, #58965, #255866 ) ;
#84585=ORIENTED_EDGE ( 'NONE', *, *, #28727, .T. ) ;
#84740=EDGE_LOOP ( 'NONE', ( #249623, #164495, #128162, #224919 ) ) ;
#84830=CARTESIAN_POINT ( 'NONE',  ( -13.77178122865954180, 9.456028260507913785, -15.01119803506572659 ) ) ;
#85243=EDGE_CURVE ( 'NONE', #43971, #118880, #96172, .T. ) ;
#85297=CARTESIAN_POINT ( 'NONE',  ( -18.35668295345803713, 11.47316190336247388, -24.25000000000001066 ) ) ;
#85504=ORIENTED_EDGE ( 'NONE', *, *, #123280, .T. ) ;
#85642=EDGE_LOOP ( 'NONE', ( #46631, #81235, #176323, #249048 ) ) ;
#85715=PLANE ( 'NONE',  #257864 ) ;
#85894=CARTESIAN_POINT ( 'NONE',  ( -16.93906926870270624, 10.01214687094654998, -12.55345230722682359 ) ) ;
#85937=DIRECTION ( 'NONE',  ( 0.5932847527679310229, -0.8049926720990042694, 0.000000000000000000 ) ) ;
#85956=LINE ( 'NONE', #205935, #206919 ) ;
#85983=VECTOR ( 'NONE', #210347, 1000.000000000000000 ) ;
#86042=VERTEX_POINT ( 'NONE', #220811 ) ;
#86280=LINE ( 'NONE', #128013, #96479 ) ;
#86309=( GEOMETRIC_REPRESENTATION_CONTEXT ( 3 ) GLOBAL_UNCERTAINTY_ASSIGNED_CONTEXT ( ( #140545 ) ) GLOBAL_UNIT_ASSIGNED_CONTEXT ( ( #164712, #47299, #6912 ) ) REPRESENTATION_CONTEXT ( 'NONE', 'WORKASPACE' ) );
#86390=VERTEX_POINT ( 'NONE', #238467 ) ;
#86423=CARTESIAN_POINT ( 'NONE',  ( -16.89268316805465986, 9.951721813242182080, -20.85575247854553993 ) ) ;
#86497=VERTEX_POINT ( 'NONE', #225297 ) ;
#86689=AXIS2_PLACEMENT_3D ( 'NONE', #242746, #4143, #122834 ) ;
#86963=DIRECTION ( 'NONE',  ( -1.000000000000000000, 0.000000000000000000, 0.000000000000000000 ) ) ;
#87166=ORIENTED_EDGE ( 'NONE', *, *, #70773, .F. ) ;
#87507=CARTESIAN_POINT ( 'NONE',  ( 13.99999999999999822, 9.849999999999981881, -16.74999999999999645 ) ) ;
#87671=ORIENTED_EDGE ( 'NONE', *, *, #128569, .T. ) ;
#87791=DIRECTION ( 'NONE',  ( -0.000000000000000000, -0.000000000000000000, -1.000000000000000000 ) ) ;
#87942=EDGE_CURVE ( 'NONE', #14615, #12920, #231530, .T. ) ;
#87992=FACE_OUTER_BOUND ( 'NONE', #177112, .T. ) ;
#88069=DIRECTION ( 'NONE',  ( 0.000000000000000000, 0.9553114395362829470, -0.2956011730205325705 ) ) ;
#88133=CARTESIAN_POINT ( 'NONE',  ( -16.94389599338512298, 9.991197989755043807, -12.60764480181024538 ) ) ;
#88276=ORIENTED_EDGE ( 'NONE', *, *, #89002, .F. ) ;
#88381=CARTESIAN_POINT ( 'NONE',  ( -16.88460203013675454, 9.954759003235713166, -20.86589180953822975 ) ) ;
#88402=VERTEX_POINT ( 'NONE', #217028 ) ;
#88468=CARTESIAN_POINT ( 'NONE',  ( -16.93772744219066340, 9.993541108752353352, -12.59806197196970068 ) ) ;
#88580=FACE_OUTER_BOUND ( 'NONE', #142747, .T. ) ;
#88756=VERTEX_POINT ( 'NONE', #98042 ) ;
#88871=FACE_OUTER_BOUND ( 'NONE', #206775, .T. ) ;
#89002=EDGE_CURVE ( 'NONE', #50885, #248097, #242260, .T. ) ;
#89038=FACE_OUTER_BOUND ( 'NONE', #47838, .T. ) ;
#89143=CARTESIAN_POINT ( 'NONE',  ( 14.45963434102923983, 9.451541661385506998, -18.45387549883058398 ) ) ;
#89182=EDGE_CURVE ( 'NONE', #82768, #60760, #228836, .T. ) ;
#89418=CARTESIAN_POINT ( 'NONE',  ( 18.39999999999998082, 11.47316190336247033, -9.250000000000000000 ) ) ;
#89614=CARTESIAN_POINT ( 'NONE',  ( 21.13736287352038445, 8.046642376383999817, -12.65000000000000568 ) ) ;
#89720=STYLED_ITEM ( 'NONE', ( #79075 ), #144531 ) ;
#89744=( BOUNDED_CURVE ( )  B_SPLINE_CURVE ( 3, ( #204617, #166829, #44289, #145930 ),
 .UNSPECIFIED., .F., .F. ) 
 B_SPLINE_CURVE_WITH_KNOTS ( ( 4, 4 ),
 ( 3.752122642744643688, 4.712388980384671910 ),
 .UNSPECIFIED. ) 
 CURVE ( )  GEOMETRIC_REPRESENTATION_ITEM ( )  RATIONAL_B_SPLINE_CURVE ( ( 1.000000000000000000, 0.9246222802177312960, 0.9246222802177312960, 1.000000000000000000 ) ) 
 REPRESENTATION_ITEM ( '' )  );
#89765=CARTESIAN_POINT ( 'NONE',  ( -16.93583594267724379, 10.00862343505220053, -12.55939083932076272 ) ) ;
#89767=CARTESIAN_POINT ( 'NONE',  ( 21.72449340488910252, 10.28395627749112151, -12.65000000000000568 ) ) ;
#90030=EDGE_CURVE ( 'NONE', #96167, #200257, #11901, .T. ) ;
#90094=EDGE_CURVE ( 'NONE', #191176, #209877, #135010, .T. ) ;
#90112=CARTESIAN_POINT ( 'NONE',  ( -17.04761207306819770, 10.02645087339777241, -12.65000000000000213 ) ) ;
#90148=CARTESIAN_POINT ( 'NONE',  ( 23.04999999999999716, 8.822561741666397950, -9.250000000000001776 ) ) ;
#90422=CARTESIAN_POINT ( 'NONE',  ( 12.42718393586866554, 9.370655051123481627, -17.52582325598087820 ) ) ;
#90468=EDGE_CURVE ( 'NONE', #196735, #163267, #256449, .T. ) ;
#90521=ORIENTED_EDGE ( 'NONE', *, *, #244267, .F. ) ;
#90923=FACE_OUTER_BOUND ( 'NONE', #221137, .T. ) ;
#91101=CARTESIAN_POINT ( 'NONE',  ( 18.39999999999999503, 11.47316190336248454, -12.65000000000000213 ) ) ;
#91210=ORIENTED_EDGE ( 'NONE', *, *, #186769, .T. ) ;
#91386=EDGE_CURVE ( 'NONE', #51112, #201670, #176473, .T. ) ;
#91719=CARTESIAN_POINT ( 'NONE',  ( -16.83233564386404879, 9.930221796584600469, -12.77547933652440726 ) ) ;
#91722=CARTESIAN_POINT ( 'NONE',  ( 12.84435279558019793, 9.410708747047079825, -18.06920840584410115 ) ) ;
#91778=CARTESIAN_POINT ( 'NONE',  ( -16.90138253750127006, 9.949999999999983302, -20.71156270790459075 ) ) ;
#91942=CARTESIAN_POINT ( 'NONE',  ( -21.64999999999999858, 9.349999999999978328, -9.250000000000001776 ) ) ;
#92111=ORIENTED_EDGE ( 'NONE', *, *, #231915, .F. ) ;
#92249=CARTESIAN_POINT ( 'NONE',  ( -16.81744102076748959, 9.949999999999983302, -20.85000000000000142 ) ) ;
#92407=DIRECTION ( 'NONE',  ( -0.000000000000000000, 1.000000000000000000, -0.000000000000000000 ) ) ;
#92740=VERTEX_POINT ( 'NONE', #2434 ) ;
#92895=ORIENTED_EDGE ( 'NONE', *, *, #67308, .T. ) ;
#93002=CARTESIAN_POINT ( 'NONE',  ( 13.43663047529819821, 9.446645344695243196, -18.41080645610018607 ) ) ;
#93121=CARTESIAN_POINT ( 'NONE',  ( -12.25000000000000178, 9.849999999999978328, -16.75000000000000355 ) ) ;
#93135=ORIENTED_EDGE ( 'NONE', *, *, #13020, .F. ) ;
#93149=DIRECTION ( 'NONE',  ( -0.000000000000000000, -0.000000000000000000, -1.000000000000000000 ) ) ;
#93198=DIRECTION ( 'NONE',  ( -1.000000000000000000, -1.186688945009010077E-16, -0.000000000000000000 ) ) ;
#93234=FACE_OUTER_BOUND ( 'NONE', #60528, .T. ) ;
#93447=CARTESIAN_POINT ( 'NONE',  ( -16.93589915522259304, 10.00862525869585617, -20.94056010196031181 ) ) ;
#93504=ORIENTED_EDGE ( 'NONE', *, *, #25035, .F. ) ;
#93546=ORIENTED_EDGE ( 'NONE', *, *, #233760, .T. ) ;
#93963=CARTESIAN_POINT ( 'NONE',  ( -16.92507428761701505, 9.949999999999983302, -12.71339745962155909 ) ) ;
#94382=PLANE ( 'NONE',  #186982 ) ;
#94384=CARTESIAN_POINT ( 'NONE',  ( 20.73486653747088582, 7.250000000000026645, -20.85000000000000142 ) ) ;
#94554=CARTESIAN_POINT ( 'NONE',  ( -18.34804628011471195, 11.47316190336237796, -9.250000000000001776 ) ) ;
#94627=DIRECTION ( 'NONE',  ( 1.000000000000000000, 0.000000000000000000, 0.000000000000000000 ) ) ;
#94715=AXIS2_PLACEMENT_3D ( 'NONE', #182119, #157453, #43888 ) ;
#94860=EDGE_CURVE ( 'NONE', #7235, #140173, #124041, .T. ) ;
#94914=CIRCLE ( 'NONE', #219811, 0.9000000000000014655 ) ;
#94940=CARTESIAN_POINT ( 'NONE',  ( -16.83199030136657726, 9.930648033113465445, -12.77240102265748156 ) ) ;
#94977=CARTESIAN_POINT ( 'NONE',  ( -18.40000000000000213, 5.649999999999983480, -20.85000000000000142 ) ) ;
#95294=VERTEX_POINT ( 'NONE', #121558 ) ;
#95450=CARTESIAN_POINT ( 'NONE',  ( -15.55912972643741199, 8.490870273562562076, -12.55000000000000249 ) ) ;
#95513=CARTESIAN_POINT ( 'NONE',  ( -16.91776028072577631, 9.963400393629743945, -20.87502401470212732 ) ) ;
#95526=CARTESIAN_POINT ( 'NONE',  ( -14.00000000000000178, 9.849999999999978328, -16.75000000000000355 ) ) ;
#95590=AXIS2_PLACEMENT_3D ( 'NONE', #73782, #34650, #253655 ) ;
#95957=CARTESIAN_POINT ( 'NONE',  ( -23.25000000000000355, 9.949999999999983302, -9.250000000000001776 ) ) ;
#95976=ORIENTED_EDGE ( 'NONE', *, *, #71892, .T. ) ;
#96006=VECTOR ( 'NONE', #246870, 1000.000000000000000 ) ;
#96013=CARTESIAN_POINT ( 'NONE',  ( -16.93415306273742260, 9.995622260012515525, -20.91005694236041634 ) ) ;
#96109=ORIENTED_EDGE ( 'NONE', *, *, #167386, .T. ) ;
#96167=VERTEX_POINT ( 'NONE', #149475 ) ;
#96172=LINE ( 'NONE', #160041, #13289 ) ;
#96345=AXIS2_PLACEMENT_3D ( 'NONE', #154535, #157080, #234025 ) ;
#96432=DIRECTION ( 'NONE',  ( 1.000000000000000000, 0.000000000000000000, 0.000000000000000000 ) ) ;
#96479=VECTOR ( 'NONE', #68028, 1000.000000000000000 ) ;
#96520=CARTESIAN_POINT ( 'NONE',  ( -16.97683809663752186, 9.949999999999983302, -13.40236401819648648 ) ) ;
#96806=CYLINDRICAL_SURFACE ( 'NONE', #84476, 0.9000000000000014655 ) ;
#96938=AXIS2_PLACEMENT_3D ( 'NONE', #33275, #93198, #9814 ) ;
#97034=CARTESIAN_POINT ( 'NONE',  ( 14.77516762759922031, 9.436674251842843475, -15.17686193099920722 ) ) ;
#97085=CARTESIAN_POINT ( 'NONE',  ( 21.72449340488910252, 10.28395627749112151, -12.65000000000000568 ) ) ;
#97468=DIRECTION ( 'NONE',  ( -0.7071067811865562325, -0.7071067811865388020, 0.000000000000000000 ) ) ;
#97863=PRODUCT_DEFINITION ( 'UNKNOWN', '', #61421, #212352 ) ;
#97942=ORIENTED_EDGE ( 'NONE', *, *, #127937, .T. ) ;
#98042=CARTESIAN_POINT ( 'NONE',  ( 21.13736287352038445, 8.046642376383999817, -20.84999999999999787 ) ) ;
#98552=PLANE ( 'NONE',  #73798 ) ;
#98615=VECTOR ( 'NONE', #33644, 1000.000000000000000 ) ;
#98653=CARTESIAN_POINT ( 'NONE',  ( -16.89318236219976654, 9.951535257875130824, -12.64487036789414276 ) ) ;
#98684=AXIS2_PLACEMENT_3D ( 'NONE', #202, #75900, #155478 ) ;
#98803=EDGE_LOOP ( 'NONE', ( #185090, #217722, #167026 ) ) ;
#99122=CARTESIAN_POINT ( 'NONE',  ( -16.87036670365549540, 9.989418819301647545, -12.52043988269794106 ) ) ;
#99249=EDGE_CURVE ( 'NONE', #35963, #248097, #181107, .T. ) ;
#99288=FACE_OUTER_BOUND ( 'NONE', #142929, .T. ) ;
#99290=CARTESIAN_POINT ( 'NONE',  ( -16.94107738177414291, 10.01423928513661465, -20.94999999999998863 ) ) ;
#99369=ORIENTED_EDGE ( 'NONE', *, *, #40903, .T. ) ;
#99402=EDGE_LOOP ( 'NONE', ( #250309, #77645, #50218, #152859, #240092, #171192, #91210, #25524, #112047, #121648, #123975, #245559, #120181, #163690, #206617, #93504, #145436, #102802 ) ) ;
#99553=B_SPLINE_CURVE_WITH_KNOTS ( 'NONE', 3,
 ( #233860, #55176, #10962, #213003, #91778, #134732, #132189, #53933, #170078, #31835 ),
 .UNSPECIFIED., .F., .F.,
 ( 4, 2, 2, 2, 4 ),
 ( 5.280516497093958406E-16, 9.930191194499918771E-05, 0.0001986038238894703419, 0.0003972076477784197246, 0.0007944152955563271636 ),
 .UNSPECIFIED. ) ;
#99696=CARTESIAN_POINT ( 'NONE',  ( -16.87683809663752399, 9.865889849332424077, -20.23257319293034939 ) ) ;
#99701=CARTESIAN_POINT ( 'NONE',  ( -16.77683809663752257, 9.945835743204147761, -20.83605098089580210 ) ) ;
#100001=DIRECTION ( 'NONE',  ( 1.000000000000000000, 0.000000000000000000, 0.000000000000000000 ) ) ;
#100236=CARTESIAN_POINT ( 'NONE',  ( 18.54999999999999716, 9.949999999999997513, -12.64999999999994529 ) ) ;
#100450=AXIS2_PLACEMENT_3D ( 'NONE', #18310, #220376, #256868 ) ;
#100562=CARTESIAN_POINT ( 'NONE',  ( -18.44085059012131822, 11.51401249348380063, -24.24030531912154629 ) ) ;
#100742=ORIENTED_EDGE ( 'NONE', *, *, #167510, .T. ) ;
#100847=DIRECTION ( 'NONE',  ( -1.020425574104004196E-15, -1.210927747993693964E-31, -1.000000000000000000 ) ) ;
#100984=CARTESIAN_POINT ( 'NONE',  ( -18.40000000000000213, 11.48667500175767131, -24.25000000000000000 ) ) ;
#101084=ADVANCED_FACE ( 'NONE', ( #113833 ), #96806, .F. ) ;
#101212=VERTEX_POINT ( 'NONE', #220649 ) ;
#101316=VECTOR ( 'NONE', #123618, 1000.000000000000000 ) ;
#101325=ORIENTED_EDGE ( 'NONE', *, *, #221688, .T. ) ;
#101380=EDGE_CURVE ( 'NONE', #163267, #106852, #170987, .T. ) ;
#101603=FACE_BOUND ( 'NONE', #108552, .T. ) ;
#101673=LINE ( 'NONE', #144671, #181146 ) ;
#102040=DIRECTION ( 'NONE',  ( -0.000000000000000000, 1.000000000000000000, -0.000000000000000000 ) ) ;
#102084=ORIENTED_EDGE ( 'NONE', *, *, #147422, .T. ) ;
#102252=CARTESIAN_POINT ( 'NONE',  ( -16.79184697841823848, 9.948761661658393152, -12.65414227060253083 ) ) ;
#102737=ORIENTED_EDGE ( 'NONE', *, *, #94860, .F. ) ;
#102802=ORIENTED_EDGE ( 'NONE', *, *, #163025, .T. ) ;
#102853=EDGE_CURVE ( 'NONE', #208072, #200257, #101673, .T. ) ;
#102925=CARTESIAN_POINT ( 'NONE',  ( -14.87770893841227071, 9.430637101696738966, -18.26826061806095325 ) ) ;
#102957=CARTESIAN_POINT ( 'NONE',  ( 18.54999999999999716, 9.949999999999997513, -20.85000000000005471 ) ) ;
#102999=ORIENTED_EDGE ( 'NONE', *, *, #32846, .F. ) ;
#103099=ORIENTED_EDGE ( 'NONE', *, *, #90468, .T. ) ;
#103129=CARTESIAN_POINT ( 'NONE',  ( -13.12432614554022869, 9.430764995422318719, -15.23053739475045987 ) ) ;
#103278=AXIS2_PLACEMENT_3D ( 'NONE', #56757, #94627, #215846 ) ;
#103378=CARTESIAN_POINT ( 'NONE',  ( -16.77683809663752257, 23.65833333333332433, -16.75000000000000000 ) ) ;
#103555=CARTESIAN_POINT ( 'NONE',  ( -16.87401514999228525, 9.949999999999983302, -20.78001799253221193 ) ) ;
#103725=B_SPLINE_CURVE_WITH_KNOTS ( 'NONE', 3,
 ( #49475, #67755, #187723, #226823 ),
 .UNSPECIFIED., .F., .F.,
 ( 4, 4 ),
 ( 0.000000000000000000, 7.713889350929744009E-05 ),
 .UNSPECIFIED. ) ;
#103840=DIRECTION ( 'NONE',  ( 1.000000000000000000, 0.000000000000000000, 0.000000000000000000 ) ) ;
#103972=CARTESIAN_POINT ( 'NONE',  ( -16.88815647973234135, 9.950832619315736594, -12.64721706332599638 ) ) ;
#104014=CARTESIAN_POINT ( 'NONE',  ( -16.94107738177414291, 10.01423928513661821, -20.94999999999999929 ) ) ;
#104169=ORIENTED_EDGE ( 'NONE', *, *, #163323, .T. ) ;
#104177=VECTOR ( 'NONE', #227714, 999.9999999999998863 ) ;
#104416=LINE ( 'NONE', #23659, #172035 ) ;
#104930=CARTESIAN_POINT ( 'NONE',  ( -16.80939487329394666, 9.949999999999983302, -20.85000000000088249 ) ) ;
#105000=ORIENTED_EDGE ( 'NONE', *, *, #91386, .T. ) ;
#105106=CARTESIAN_POINT ( 'NONE',  ( -33.72168855820452649, 11.47316190336247388, -24.25000000000001066 ) ) ;
#105337=ORIENTED_EDGE ( 'NONE', *, *, #21154, .T. ) ;
#105453=CARTESIAN_POINT ( 'NONE',  ( -16.93339986808596720, 10.00510392856591757, -12.56599367181285487 ) ) ;
#105478=CARTESIAN_POINT ( 'NONE',  ( -12.42749937872396515, 9.370689921602609829, -17.52646512666106204 ) ) ;
#105691=ORIENTED_EDGE ( 'NONE', *, *, #114198, .F. ) ;
#105804=EDGE_CURVE ( 'NONE', #45065, #146218, #76165, .T. ) ;
#105841=MANIFOLD_SOLID_BREP ( 'Stock-MAS-200-1', #136645 ) ;
#105908=EDGE_CURVE ( 'NONE', #203977, #14615, #202547, .T. ) ;
#106316=EDGE_CURVE ( 'NONE', #222282, #134996, #39471, .T. ) ;
#106685=VERTEX_POINT ( 'NONE', #92249 ) ;
#106852=VERTEX_POINT ( 'NONE', #156119 ) ;
#106948=CARTESIAN_POINT ( 'NONE',  ( -17.01825945287482966, 10.04999999999998295, -12.65000000000000213 ) ) ;
#107082=ORIENTED_EDGE ( 'NONE', *, *, #20595, .T. ) ;
#107156=AXIS2_PLACEMENT_3D ( 'NONE', #90148, #146281, #8080 ) ;
#107427=CARTESIAN_POINT ( 'NONE',  ( 15.39170923737819940, 9.389529397466734650, -17.81710791289368245 ) ) ;
#107428=CARTESIAN_POINT ( 'NONE',  ( -16.80070461187907682, 9.949999999999985079, -20.85303617083875238 ) ) ;
#107585=ORIENTED_EDGE ( 'NONE', *, *, #132738, .T. ) ;
#107591=ORIENTED_EDGE ( 'NONE', *, *, #223648, .F. ) ;
#107668=DIRECTION ( 'NONE',  ( 0.000000000000000000, 0.000000000000000000, -1.000000000000000000 ) ) ;
#107712=AXIS2_PLACEMENT_3D ( 'NONE', #194084, #209779, #54545 ) ;
#107846=CARTESIAN_POINT ( 'NONE',  ( -16.89268316805466341, 9.951721813242185632, -12.64424752145445296 ) ) ;
#108313=DIRECTION ( 'NONE',  ( 1.020425574104004196E-15, 1.210927747993693964E-31, 1.000000000000000000 ) ) ;
#108552=EDGE_LOOP ( 'NONE', ( #233632, #58499 ) ) ;
#108718=CARTESIAN_POINT ( 'NONE',  ( 15.07585980824112859, 9.417632963106287391, -18.14894846573225706 ) ) ;
#108735=ORIENTED_EDGE ( 'NONE', *, *, #204584, .T. ) ;
#108790=ORIENTED_EDGE ( 'NONE', *, *, #40903, .F. ) ;
#108864=DIRECTION ( 'NONE',  ( -1.020425574104004196E-15, 0.000000000000000000, 1.000000000000000000 ) ) ;
#109071=VERTEX_POINT ( 'NONE', #82951 ) ;
#109150=EDGE_CURVE ( 'NONE', #5409, #28990, #252313, .T. ) ;
#109343=CARTESIAN_POINT ( 'NONE',  ( -15.06720934482788365, 9.417690691063098640, -18.14160069676458420 ) ) ;
#109456=EDGE_CURVE ( 'NONE', #17161, #35963, #167383, .T. ) ;
#109459=ORIENTED_EDGE ( 'NONE', *, *, #182872, .F. ) ;
#109562=EDGE_LOOP ( 'NONE', ( #113655, #164775, #134728, #121056, #241642, #53645, #107082, #235034, #46994 ) ) ;
#109712=EDGE_CURVE ( 'NONE', #158579, #195135, #36866, .T. ) ;
#109917=FACE_OUTER_BOUND ( 'NONE', #239032, .T. ) ;
#110112=CARTESIAN_POINT ( 'NONE',  ( -17.78043020864320667, 10.85359211200568375, -10.33695083427979178 ) ) ;
#110164=CARTESIAN_POINT ( 'NONE',  ( -23.25000000000000355, 11.74999999999998224, -20.85000000000000142 ) ) ;
#110286=( BOUNDED_CURVE ( )  B_SPLINE_CURVE ( 3, ( #241546, #139860, #122896, #164587 ),
 .UNSPECIFIED., .F., .F. ) 
 B_SPLINE_CURVE_WITH_KNOTS ( ( 4, 4 ),
 ( 3.432212674861196966, 3.693332928900581624 ),
 .UNSPECIFIED. ) 
 CURVE ( )  GEOMETRIC_REPRESENTATION_ITEM ( )  RATIONAL_B_SPLINE_CURVE ( ( 1.000000000000000000, 0.9943260843901261525, 0.9943260843901261525, 1.000000000000000000 ) ) 
 REPRESENTATION_ITEM ( '' )  );
#110332=ORIENTED_EDGE ( 'NONE', *, *, #198586, .F. ) ;
#110473=B_SPLINE_CURVE_WITH_KNOTS ( 'NONE', 3,
 ( #125094, #122526, #204601, #25989, #1259, #105478, #185048, #6408, #119981, #142062, #199503, #221585, #80790, #160386, #161665, #42983, #202054, #23445, #102925, #109343, #169385, #67668, #190200, #10281, #229327, #187640, #250166, #228032, #147206, #186349 ),
 .UNSPECIFIED., .F., .F.,
 ( 4, 2, 2, 2, 2, 2, 2, 2, 2, 2, 2, 2, 2, 2, 4 ),
 ( 0.000000000000000000, 0.0003422764154113400658, 0.0006845528308226801317, 0.001026829246234020306, 0.001369105661645360263, 0.002053658492468029336, 0.002738211323290697975, 0.003080487738702029476, 0.003422764154113361410, 0.003765040569524692477, 0.004107316984936024845, 0.004449593400347355912, 0.004791869815758687846, 0.005134146231170023250, 0.005476422646581358654 ),
 .UNSPECIFIED. ) ;
#110496=DIRECTION ( 'NONE',  ( -1.020425574104004196E-15, -0.000000000000000000, -1.000000000000000000 ) ) ;
#110625=CARTESIAN_POINT ( 'NONE',  ( -16.94037747912386394, 10.01353938248632858, -12.55113095797549327 ) ) ;
#110992=AXIS2_PLACEMENT_3D ( 'NONE', #144267, #244667, #100001 ) ;
#111211=CARTESIAN_POINT ( 'NONE',  ( 22.88900146558018989, 8.703904791112817563, -12.65000000000000746 ) ) ;
#111251=ORIENTED_EDGE ( 'NONE', *, *, #167386, .F. ) ;
#111287=CARTESIAN_POINT ( 'NONE',  ( -16.80891096016323516, 9.949999999999983302, -12.63233719273114275 ) ) ;
#111292=CARTESIAN_POINT ( 'NONE',  ( 12.48201962039795987, 9.376659938533533634, -17.62819254821727100 ) ) ;
#111406=CARTESIAN_POINT ( 'NONE',  ( -17.29158576265544056, 10.36474766601791409, -11.41724175520783113 ) ) ;
#111686=CARTESIAN_POINT ( 'NONE',  ( -16.87036670365548474, 9.989418819301645769, -20.97956011730205006 ) ) ;
#111795=LINE ( 'NONE', #33583, #122724 ) ;
#111812=DIRECTION ( 'NONE',  ( 0.000000000000000000, 0.000000000000000000, 1.000000000000000000 ) ) ;
#111833=CARTESIAN_POINT ( 'NONE',  ( -16.86733706339143524, 9.965990529639665141, -20.90311530199869949 ) ) ;
#112041=DIRECTION ( 'NONE',  ( 1.000000000000000000, 0.000000000000000000, 0.000000000000000000 ) ) ;
#112047=ORIENTED_EDGE ( 'NONE', *, *, #255705, .T. ) ;
#112128=AXIS2_PLACEMENT_3D ( 'NONE', #83864, #248116, #68206 ) ;
#112372=EDGE_LOOP ( 'NONE', ( #150343, #85504, #6991, #60537 ) ) ;
#112465=DIRECTION ( 'NONE',  ( 0.7071067811865474617, 0.7071067811865474617, 0.000000000000000000 ) ) ;
#112577=CARTESIAN_POINT ( 'NONE',  ( -16.84793658983432607, 9.949999999999985079, -12.73364667781021708 ) ) ;
#112669=EDGE_LOOP ( 'NONE', ( #169553, #132545, #129730, #148360 ) ) ;
#112699=LINE ( 'NONE', #93121, #13882 ) ;
#113074=DIRECTION ( 'NONE',  ( -1.000000000000000000, 0.000000000000000000, 0.000000000000000000 ) ) ;
#113547=CIRCLE ( 'NONE', #96938, 14.20833333333333748 ) ;
#113655=ORIENTED_EDGE ( 'NONE', *, *, #194510, .T. ) ;
#113833=FACE_OUTER_BOUND ( 'NONE', #112669, .T. ) ;
#114091=DIRECTION ( 'NONE',  ( -1.000000000000000000, 0.000000000000000000, 0.000000000000000000 ) ) ;
#114118=CARTESIAN_POINT ( 'NONE',  ( -18.35663730107557257, 11.47390742651120021, -9.250000000000001776 ) ) ;
#114198=EDGE_CURVE ( 'NONE', #195203, #60760, #71191, .T. ) ;
#114283=LINE ( 'NONE', #170461, #13083 ) ;
#114379=( NAMED_UNIT ( * ) PLANE_ANGLE_UNIT ( ) SI_UNIT ( $, .RADIAN. ) );
#114519=CARTESIAN_POINT ( 'NONE',  ( -18.40000000000000213, 11.48667500175766953, -9.250000000000001776 ) ) ;
#114858=ORIENTED_EDGE ( 'NONE', *, *, #191807, .F. ) ;
#114881=AXIS2_PLACEMENT_3D ( 'NONE', #140852, #220395, #48155 ) ;
#115010=CARTESIAN_POINT ( 'NONE',  ( 23.24999999999999645, 11.74999999999998224, -12.65000000000000746 ) ) ;
#115084=CARTESIAN_POINT ( 'NONE',  ( -16.94445028196807002, 9.992063609697737547, -20.89266982158155628 ) ) ;
#115214=FACE_OUTER_BOUND ( 'NONE', #21962, .T. ) ;
#115619=AXIS2_PLACEMENT_3D ( 'NONE', #87507, #125378, #143641 ) ;
#115738=CARTESIAN_POINT ( 'NONE',  ( -18.39999999999999858, 11.47316190336248631, -20.89142135623730212 ) ) ;
#115788=TOROIDAL_SURFACE ( 'NONE', #119923, 14.20833333333334103, 0.1000000000000000056 ) ;
#115867=CARTESIAN_POINT ( 'NONE',  ( -17.11825945287482753, 9.949999999999983302, -12.65000000000000213 ) ) ;
#116110=EDGE_CURVE ( 'NONE', #225349, #254638, #139282, .T. ) ;
#116152=ORIENTED_EDGE ( 'NONE', *, *, #35996, .F. ) ;
#116233=VERTEX_POINT ( 'NONE', #246120 ) ;
#116305=CARTESIAN_POINT ( 'NONE',  ( 18.39999999999999503, 11.47316190336248454, -12.65000000000000213 ) ) ;
#116435=ORIENTED_EDGE ( 'NONE', *, *, #227411, .F. ) ;
#116530=AXIS2_PLACEMENT_3D ( 'NONE', #25572, #180793, #127230 ) ;
#116645=CARTESIAN_POINT ( 'NONE',  ( 13.76927104934457624, 9.455987233612738407, -15.01153116689782507 ) ) ;
#117007=VECTOR ( 'NONE', #125052, 1000.000000000000000 ) ;
#117021=CARTESIAN_POINT ( 'NONE',  ( -18.40000000000000213, 11.47316190336248809, -20.94999999999999929 ) ) ;
#117090=CARTESIAN_POINT ( 'NONE',  ( -16.87372386987899375, 9.880600233636760876, -13.14926987186641405 ) ) ;
#117657=DIRECTION ( 'NONE',  ( 1.000000000000000000, 1.186688945009010077E-16, 0.000000000000000000 ) ) ;
#117729=EDGE_LOOP ( 'NONE', ( #137136, #190479, #132275, #140600, #14701 ) ) ;
#117748=CARTESIAN_POINT ( 'NONE',  ( -16.94107738177414291, 10.01423928513661998, -20.94999999999999929 ) ) ;
#117782=DIRECTION ( 'NONE',  ( -1.000000000000000000, 0.000000000000000000, 0.000000000000000000 ) ) ;
#117870=CARTESIAN_POINT ( 'NONE',  ( -16.88853107394619357, 9.950878483346977887, -20.85293634689222841 ) ) ;
#117908=ORIENTED_EDGE ( 'NONE', *, *, #170786, .F. ) ;
#118017=ORIENTED_EDGE ( 'NONE', *, *, #226076, .F. ) ;
#118698=CARTESIAN_POINT ( 'NONE',  ( -16.97048326478264713, 9.949999999999983302, -13.14110688012716999 ) ) ;
#118880=VERTEX_POINT ( 'NONE', #115010 ) ;
#118899=CARTESIAN_POINT ( 'NONE',  ( -17.29838795458705647, 10.37154985794953177, -22.10474128261738613 ) ) ;
#118991=CIRCLE ( 'NONE', #114881, 0.09999999999999939493 ) ;
#119044=ORIENTED_EDGE ( 'NONE', *, *, #139800, .T. ) ;
#119296=CARTESIAN_POINT ( 'NONE',  ( -16.81095280782811230, 9.949999999999983302, -12.64999999999912639 ) ) ;
#119298=CARTESIAN_POINT ( 'NONE',  ( -16.87683809663752399, 9.849999999999983658, -20.09763598180368405 ) ) ;
#119675=VECTOR ( 'NONE', #137420, 1000.000000000000000 ) ;
#119923=AXIS2_PLACEMENT_3D ( 'NONE', #103378, #199956, #237783 ) ;
#119981=CARTESIAN_POINT ( 'NONE',  ( -12.68215100488889924, 9.396630376317714806, -17.90705739281830589 ) ) ;
#120028=CARTESIAN_POINT ( 'NONE',  ( -16.94107738177415357, 10.01423928513661998, -12.54999999999999361 ) ) ;
#120181=ORIENTED_EDGE ( 'NONE', *, *, #180100, .T. ) ;
#120279=VECTOR ( 'NONE', #245001, 1000.000000000000000 ) ;
#120285=CARTESIAN_POINT ( 'NONE',  ( -18.40000000000000213, 11.47316190336248809, -24.17405393319204876 ) ) ;
#120391=CYLINDRICAL_SURFACE ( 'NONE', #47194, 0.09999999999999939493 ) ;
#120478=FILL_AREA_STYLE ('',( #237823 ) ) ;
#120598=CARTESIAN_POINT ( 'NONE',  ( -16.89935556175703368, 9.949999999999985079, -20.36032363711476734 ) ) ;
#120862=CARTESIAN_POINT ( 'NONE',  ( -16.92570016628984675, 9.958788957739859171, -12.62065067003899088 ) ) ;
#120924=FACE_OUTER_BOUND ( 'NONE', #169168, .T. ) ;
#120973=ADVANCED_FACE ( 'NONE', ( #9888 ), #169014, .T. ) ;
#121056=ORIENTED_EDGE ( 'NONE', *, *, #209129, .F. ) ;
#121462=CARTESIAN_POINT ( 'NONE',  ( -14.23072895065543264, 9.455987233612740184, -15.01153116689783040 ) ) ;
#121558=CARTESIAN_POINT ( 'NONE',  ( -18.40000000000000213, 11.33174054712517886, -20.85000000000000142 ) ) ;
#121648=ORIENTED_EDGE ( 'NONE', *, *, #24938, .T. ) ;
#122043=EDGE_CURVE ( 'NONE', #68437, #47344, #176452, .T. ) ;
#122065=CARTESIAN_POINT ( 'NONE',  ( -23.25000000000000355, 5.649999999999983480, -20.85000000000000142 ) ) ;
#122070=VECTOR ( 'NONE', #62346, 1000.000000000000000 ) ;
#122121=CARTESIAN_POINT ( 'NONE',  ( -16.92973740335356680, 9.992503814467269763, -12.59394096479777048 ) ) ;
#122526=CARTESIAN_POINT ( 'NONE',  ( -12.25000000000000355, 9.349999999999981881, -16.86574316727392286 ) ) ;
#122566=VECTOR ( 'NONE', #202134, 1000.000000000000000 ) ;
#122644=ORIENTED_EDGE ( 'NONE', *, *, #16707, .F. ) ;
#122724=VECTOR ( 'NONE', #113074, 1000.000000000000000 ) ;
#122735=CARTESIAN_POINT ( 'NONE',  ( -14.11697426661281618, 9.457410944767410399, -15.00008397379002822 ) ) ;
#122834=DIRECTION ( 'NONE',  ( 1.000000000000000000, 0.000000000000000000, 0.000000000000000000 ) ) ;
#122896=CARTESIAN_POINT ( 'NONE',  ( 17.74533788810829904, 10.81849979147079210, -23.18637732505242610 ) ) ;
#123280=EDGE_CURVE ( 'NONE', #96167, #116233, #162054, .T. ) ;
#123352=CARTESIAN_POINT ( 'NONE',  ( 18.54999999999999716, 8.750000000000024869, -12.65000000000000213 ) ) ;
#123618=DIRECTION ( 'NONE',  ( -0.000000000000000000, -0.000000000000000000, -1.000000000000000000 ) ) ;
#123754=DIRECTION ( 'NONE',  ( -1.000000000000000000, 0.000000000000000000, 1.927470528863115795E-15 ) ) ;
#123784=CARTESIAN_POINT ( 'NONE',  ( -33.72168855820452649, 23.65833333333332433, -16.75000000000000000 ) ) ;
#123975=ORIENTED_EDGE ( 'NONE', *, *, #182377, .T. ) ;
#124041=CIRCLE ( 'NONE', #19983, 1.500000000000001332 ) ;
#124157=CIRCLE ( 'NONE', #228386, 0.5000000000000004441 ) ;
#124179=CARTESIAN_POINT ( 'NONE',  ( 18.39999999999999503, 5.649999999999983480, -12.65000000000000213 ) ) ;
#124420=DIRECTION ( 'NONE',  ( -0.000000000000000000, -0.000000000000000000, -1.000000000000000000 ) ) ;
#124611=CARTESIAN_POINT ( 'NONE',  ( -16.97683809663752186, 9.849999999999983658, -13.40236401819648648 ) ) ;
#124678=DIRECTION ( 'NONE',  ( 1.000000000000000000, 1.186688945009009831E-16, 0.000000000000000000 ) ) ;
#124718=CYLINDRICAL_SURFACE ( 'NONE', #46646, 1.749999999999999778 ) ;
#124827=CIRCLE ( 'NONE', #212331, 0.9000000000000014655 ) ;
#124846=CARTESIAN_POINT ( 'NONE',  ( -18.40000000000000213, 5.649999999999983480, -12.65000000000000213 ) ) ;
#125052=DIRECTION ( 'NONE',  ( -1.652117596168391700E-15, -1.000000000000000000, 0.000000000000000000 ) ) ;
#125067=CARTESIAN_POINT ( 'NONE',  ( -16.93970660449832621, 10.01284139163557185, -12.55228173579446960 ) ) ;
#125094=CARTESIAN_POINT ( 'NONE',  ( -12.25000000000000178, 9.349999999999983658, -16.75000000000000000 ) ) ;
#125174=ORIENTED_EDGE ( 'NONE', *, *, #51315, .F. ) ;
#125286=CARTESIAN_POINT ( 'NONE',  ( -14.56556274378147720, 9.446557523072533158, -15.08994195434589436 ) ) ;
#125378=DIRECTION ( 'NONE',  ( 1.186688945009010077E-16, -1.000000000000000000, -0.000000000000000000 ) ) ;
#125620=VERTEX_POINT ( 'NONE', #56073 ) ;
#126088=ADVANCED_FACE ( 'NONE', ( #257454 ), #239814, .F. ) ;
#126151=DIRECTION ( 'NONE',  ( -1.000000000000000000, 0.000000000000000000, 1.073024830501117725E-15 ) ) ;
#126334=CARTESIAN_POINT ( 'NONE',  ( -16.93262454970420094, 10.00202046793035571, -12.57292377376268888 ) ) ;
#126436=EDGE_CURVE ( 'NONE', #816, #86497, #153046, .T. ) ;
#126453=DIRECTION ( 'NONE',  ( 0.000000000000000000, -1.000000000000000000, 0.000000000000000000 ) ) ;
#126574=CARTESIAN_POINT ( 'NONE',  ( -16.81744102076749314, 9.949999999999986855, -12.65000000000000213 ) ) ;
#126681=DIRECTION ( 'NONE',  ( -0.000000000000000000, -0.000000000000000000, -1.000000000000000000 ) ) ;
#126788=ADVANCED_FACE ( 'NONE', ( #242465 ), #6428, .F. ) ;
#126963=CARTESIAN_POINT ( 'NONE',  ( 20.04999999999999716, 8.750000000000014211, -12.65000000000000391 ) ) ;
#126974=ORIENTED_EDGE ( 'NONE', *, *, #91386, .F. ) ;
#126995=CARTESIAN_POINT ( 'NONE',  ( 15.51872946208854920, 9.376580978043941528, -17.62694624701194002 ) ) ;
#127204=ORIENTED_EDGE ( 'NONE', *, *, #21382, .F. ) ;
#127226=DIRECTION ( 'NONE',  ( 0.000000000000000000, 0.000000000000000000, 1.000000000000000000 ) ) ;
#127230=DIRECTION ( 'NONE',  ( -1.000000000000000000, 0.000000000000000000, 0.000000000000000000 ) ) ;
#127247=ORIENTED_EDGE ( 'NONE', *, *, #24938, .F. ) ;
#127507=ADVANCED_FACE ( 'NONE', ( #189280 ), #186721, .T. ) ;
#127521=ORIENTED_EDGE ( 'NONE', *, *, #81714, .T. ) ;
#127616=EDGE_CURVE ( 'NONE', #51112, #125620, #150164, .T. ) ;
#127746=CARTESIAN_POINT ( 'NONE',  ( 15.74999999999999645, 9.349999999999983658, -16.75000000000000000 ) ) ;
#127937=EDGE_CURVE ( 'NONE', #249899, #214183, #53310, .T. ) ;
#127991=ORIENTED_EDGE ( 'NONE', *, *, #255705, .F. ) ;
#128013=CARTESIAN_POINT ( 'NONE',  ( -16.27683809663750480, 9.349999999999978328, -20.94999999999999929 ) ) ;
#128162=ORIENTED_EDGE ( 'NONE', *, *, #109150, .T. ) ;
#128290=CARTESIAN_POINT ( 'NONE',  ( 15.73863059295127798, 9.351403174141653452, -16.97953043683848762 ) ) ;
#128445=CIRCLE ( 'NONE', #249261, 0.1999999999999987899 ) ;
#128510=FACE_OUTER_BOUND ( 'NONE', #2813, .T. ) ;
#128524=PLANE ( 'NONE',  #135316 ) ;
#128559=CARTESIAN_POINT ( 'NONE',  ( 20.27550659511088682, 9.216043722508848290, -12.65000000000000391 ) ) ;
#128562=EDGE_LOOP ( 'NONE', ( #181962, #163957, #2428, #38480 ) ) ;
#128569=EDGE_CURVE ( 'NONE', #71101, #241787, #186660, .T. ) ;
#128634=VECTOR ( 'NONE', #9153, 1000.000000000000000 ) ;
#128915=CARTESIAN_POINT ( 'NONE',  ( -16.93255653858138388, 9.998451453977155623, -12.58164336798968108 ) ) ;
#129255=ORIENTED_EDGE ( 'NONE', *, *, #188004, .F. ) ;
#129297=ADVANCED_FACE ( 'NONE', ( #243543 ), #85715, .F. ) ;
#129502=CARTESIAN_POINT ( 'NONE',  ( -17.11825945287481687, 10.04999999999998472, -20.85000000000000142 ) ) ;
#129686=DIRECTION ( 'NONE',  ( 1.186688945009010077E-16, -1.000000000000000000, -0.000000000000000000 ) ) ;
#129730=ORIENTED_EDGE ( 'NONE', *, *, #244879, .T. ) ;
#129769=ADVANCED_FACE ( 'NONE', ( #87992 ), #166311, .F. ) ;
#129832=CARTESIAN_POINT ( 'NONE',  ( -14.00000000000000178, 9.849999999999978328, -16.75000000000000355 ) ) ;
#129999=CARTESIAN_POINT ( 'NONE',  ( -16.93658211146644987, 9.994108662341188776, -20.90429506995567621 ) ) ;
#130039=PLANE ( 'NONE',  #70024 ) ;
#130146=AXIS2_PLACEMENT_3D ( 'NONE', #129832, #46443, #249794 ) ;
#130175=CARTESIAN_POINT ( 'NONE',  ( -16.94062896051973865, 9.992719105100677623, -12.60251654211879924 ) ) ;
#130851=CARTESIAN_POINT ( 'NONE',  ( -21.64999999999999858, 10.04999999999998295, -20.85000000000000142 ) ) ;
#131539=ADVANCED_FACE ( 'NONE', ( #61479 ), #234444, .T. ) ;
#131599=ORIENTED_EDGE ( 'NONE', *, *, #194510, .F. ) ;
#131697=EDGE_CURVE ( 'NONE', #195203, #177395, #243957, .T. ) ;
#131811=CARTESIAN_POINT ( 'NONE',  ( -17.11825945287482753, 9.949999999999983302, -12.75000000000000178 ) ) ;
#132189=CARTESIAN_POINT ( 'NONE',  ( -16.94226253665225101, 9.949999999999983302, -20.55326540438422711 ) ) ;
#132275=ORIENTED_EDGE ( 'NONE', *, *, #48208, .T. ) ;
#132353=EDGE_CURVE ( 'NONE', #27978, #106685, #168821, .T. ) ;
#132434=VECTOR ( 'NONE', #229961, 1000.000000000000000 ) ;
#132479=ORIENTED_EDGE ( 'NONE', *, *, #29737, .T. ) ;
#132545=ORIENTED_EDGE ( 'NONE', *, *, #13020, .T. ) ;
#132680=CARTESIAN_POINT ( 'NONE',  ( -16.86379686415369150, 9.975217759253158789, -20.93338988909028231 ) ) ;
#132738=EDGE_CURVE ( 'NONE', #83518, #146218, #86280, .T. ) ;
#132814=CARTESIAN_POINT ( 'NONE',  ( -16.78493832629887450, 9.945835743204147761, -12.66394901910421567 ) ) ;
#132935=ADVANCED_FACE ( 'NONE', ( #18323 ), #162907, .T. ) ;
#133354=CARTESIAN_POINT ( 'NONE',  ( -17.11825945287481687, 9.949999999999983302, -20.75000000000000000 ) ) ;
#133640=CARTESIAN_POINT ( 'NONE',  ( 14.22821877134046886, 9.456028260507917338, -15.01119803506572659 ) ) ;
#133647=FACE_OUTER_BOUND ( 'NONE', #169762, .T. ) ;
#133964=ORIENTED_EDGE ( 'NONE', *, *, #39456, .F. ) ;
#134007=ORIENTED_EDGE ( 'NONE', *, *, #79249, .T. ) ;
#134125=CARTESIAN_POINT ( 'NONE',  ( -17.01764560440421903, 9.949999999999983302, -12.74999999921389104 ) ) ;
#134166=ORIENTED_EDGE ( 'NONE', *, *, #87942, .F. ) ;
#134262=AXIS2_PLACEMENT_3D ( 'NONE', #139541, #1311, #57436 ) ;
#134604=CARTESIAN_POINT ( 'NONE',  ( -17.05016517656120811, 9.949999999999983302, -20.82730200400101239 ) ) ;
#134672=CARTESIAN_POINT ( 'NONE',  ( -16.88705144915409306, 9.949999999999983302, -12.93097859471232525 ) ) ;
#134678=CARTESIAN_POINT ( 'NONE',  ( 12.93279065517211812, 9.417690691063100417, -18.14160069676457709 ) ) ;
#134728=ORIENTED_EDGE ( 'NONE', *, *, #229633, .F. ) ;
#134732=CARTESIAN_POINT ( 'NONE',  ( -16.92989507731676113, 9.949999999999983302, -20.61749893061018923 ) ) ;
#134823=CARTESIAN_POINT ( 'NONE',  ( -16.86578989773641979, 9.984809801258794693, -12.53533511337776574 ) ) ;
#134894=CARTESIAN_POINT ( 'NONE',  ( 12.93225390519045170, 9.417651958841004145, -15.35878739244042812 ) ) ;
#134996=VERTEX_POINT ( 'NONE', #176837 ) ;
#135010=B_SPLINE_CURVE_WITH_KNOTS ( 'NONE', 3,
 ( #96520, #78253, #118698, #255566, #1, #216489, #37882, #39167, #198208, #56112 ),
 .UNSPECIFIED., .F., .F.,
 ( 4, 2, 2, 2, 4 ),
 ( 0.000000000000000000, 0.0003916577441626798361, 0.0005874866162440179652, 0.0006854010522846884935, 0.0007833154883253590217 ),
 .UNSPECIFIED. ) ;
#135087=AXIS2_PLACEMENT_3D ( 'NONE', #34943, #12804, #175725 ) ;
#135134=CARTESIAN_POINT ( 'NONE',  ( -16.93294127766158752, 10.00328010295486081, -20.92990726582922889 ) ) ;
#135160=DIRECTION ( 'NONE',  ( 0.000000000000000000, 0.000000000000000000, 1.000000000000000000 ) ) ;
#135316=AXIS2_PLACEMENT_3D ( 'NONE', #29462, #165079, #124678 ) ;
#135328=CYLINDRICAL_SURFACE ( 'NONE', #14057, 0.1000000000000013656 ) ;
#135345=CARTESIAN_POINT ( 'NONE',  ( -16.79139129368504513, 9.944944162461677450, -12.67024463282581337 ) ) ;
#136091=ORIENTED_EDGE ( 'NONE', *, *, #183428, .F. ) ;
#136197=PLANE ( 'NONE',  #49058 ) ;
#136300=FACE_OUTER_BOUND ( 'NONE', #82901, .T. ) ;
#136348=CARTESIAN_POINT ( 'NONE',  ( 18.39999999999998082, 11.47316190336247033, -9.250000000000000000 ) ) ;
#136645=CLOSED_SHELL ( 'NONE', ( #223881, #208176, #101084, #127507, #46716, #253959, #70034, #154768, #171314, #182417, #223770, #196170, #231624, #243606, #54169, #66958, #213600, #54183, #240819, #169205, #67621, #232782, #126788, #7280, #144190, #210679, #145867, #138436, #147317, #27882, #129297, #129769, #183117, #120973, #182456, #210595, #20155, #50176, #15643, #149481, #126088, #178564, #248439, #53666, #250699, #132935, #8152, #232477, #1354, #131539, #38038, #177995, #138305 ) ) ;
#137022=CARTESIAN_POINT ( 'NONE',  ( -18.40000000000000213, 11.47316190336195341, -24.20017075153427299 ) ) ;
#137095=DIRECTION ( 'NONE',  ( 1.000000000000000000, 0.000000000000000000, -0.000000000000000000 ) ) ;
#137136=ORIENTED_EDGE ( 'NONE', *, *, #182377, .F. ) ;
#137420=DIRECTION ( 'NONE',  ( 0.000000000000000000, 0.000000000000000000, 1.000000000000000000 ) ) ;
#137473=CARTESIAN_POINT ( 'NONE',  ( 15.15590539855246455, 9.410682294267953552, -15.43114344194827581 ) ) ;
#137600=ORIENTED_EDGE ( 'NONE', *, *, #90094, .T. ) ;
#137643=DIRECTION ( 'NONE',  ( 0.000000000000000000, -0.000000000000000000, -1.000000000000000000 ) ) ;
#137757=DIRECTION ( 'NONE',  ( -0.000000000000000000, 1.000000000000000000, 0.000000000000000000 ) ) ;
#137772=FILL_AREA_STYLE_COLOUR ( '', #139589 ) ;
#137970=CARTESIAN_POINT ( 'NONE',  ( -16.92209698673604024, 9.949999999999983302, -12.71063556705198039 ) ) ;
#138249=CARTESIAN_POINT ( 'NONE',  ( -17.73285935861547813, 10.85798180378979971, -10.24143819022076052 ) ) ;
#138305=ADVANCED_FACE ( 'NONE', ( #115214 ), #120391, .T. ) ;
#138436=ADVANCED_FACE ( 'NONE', ( #2957 ), #181625, .F. ) ;
#138680=SURFACE_SIDE_STYLE ('',( #20073 ) ) ;
#138690=AXIS2_PLACEMENT_3D ( 'NONE', #153547, #233055, #111812 ) ;
#138833=VECTOR ( 'NONE', #201157, 1000.000000000000000 ) ;
#139034=( NAMED_UNIT ( * ) SI_UNIT ( $, .STERADIAN. ) SOLID_ANGLE_UNIT ( ) );
#139068=CARTESIAN_POINT ( 'NONE',  ( -16.94878442675512531, 9.991729102990998257, -12.61178042436212010 ) ) ;
#139269=AXIS2_PLACEMENT_3D ( 'NONE', #192419, #33379, #249825 ) ;
#139282=LINE ( 'NONE', #141867, #122070 ) ;
#139464=VECTOR ( 'NONE', #141788, 1000.000000000000000 ) ;
#139541=CARTESIAN_POINT ( 'NONE',  ( 18.54999999999999716, 23.65833333333332433, -16.75000000000000000 ) ) ;
#139542=EDGE_CURVE ( 'NONE', #71101, #134996, #112699, .T. ) ;
#139589=COLOUR_RGB ( '', 0.66274510, 0.83137255, 0.94901961) ;
#139724=ORIENTED_EDGE ( 'NONE', *, *, #150799, .F. ) ;
#139800=EDGE_CURVE ( 'NONE', #47766, #86497, #57768, .T. ) ;
#139860=CARTESIAN_POINT ( 'NONE',  ( 17.23472005113827166, 10.30788195450076650, -22.04657686006867578 ) ) ;
#139982=EDGE_CURVE ( 'NONE', #88756, #7969, #148877, .T. ) ;
#140060=CARTESIAN_POINT ( 'NONE',  ( -20.65000000000000568, 7.249999999999983125, -9.250000000000001776 ) ) ;
#140145=CARTESIAN_POINT ( 'NONE',  ( -18.38204789744325396, 11.47950103716508252, -24.25000000000000000 ) ) ;
#140171=ORIENTED_EDGE ( 'NONE', *, *, #250444, .F. ) ;
#140173=VERTEX_POINT ( 'NONE', #215256 ) ;
#140204=VECTOR ( 'NONE', #221060, 1000.000000000000000 ) ;
#140545=UNCERTAINTY_MEASURE_WITH_UNIT (LENGTH_MEASURE( 1.000000000000000082E-05 ), #164712, 'distance_accuracy_value', 'NONE');
#140600=ORIENTED_EDGE ( 'NONE', *, *, #221688, .F. ) ;
#140852=CARTESIAN_POINT ( 'NONE',  ( -21.64999999999999858, 10.04999999999998295, -20.75000000000000000 ) ) ;
#140980=VERTEX_POINT ( 'NONE', #242861 ) ;
#141009=CARTESIAN_POINT ( 'NONE',  ( -18.40000000000000213, 11.74999999999998224, -24.25000000000000000 ) ) ;
#141322=B_SPLINE_CURVE_WITH_KNOTS ( 'NONE', 3,
 ( #107846, #24490, #103972, #63580, #184813, #47856, #225205, #201814, #163985, #4866 ),
 .UNSPECIFIED., .F., .F.,
 ( 4, 3, 3, 4 ),
 ( 1.956645815986047257E-15, 8.145022132834093008E-06, 1.905645951092512798E-05, 2.061107371225883743E-05 ),
 .UNSPECIFIED. ) ;
#141527=DIRECTION ( 'NONE',  ( 1.000000000000000000, 0.000000000000000000, 0.000000000000000000 ) ) ;
#141580=EDGE_CURVE ( 'NONE', #181378, #214190, #38931, .T. ) ;
#141788=DIRECTION ( 'NONE',  ( -0.7071067811865463515, 0.7071067811865487940, -0.000000000000000000 ) ) ;
#141867=CARTESIAN_POINT ( 'NONE',  ( -18.40000000000000213, 11.74999999999998224, -12.65000000000000213 ) ) ;
#142048=DIRECTION ( 'NONE',  ( 0.000000000000000000, 0.000000000000000000, -1.000000000000000000 ) ) ;
#142052=CARTESIAN_POINT ( 'NONE',  ( -12.25000000000000178, 9.849999999999978328, -16.75000000000000355 ) ) ;
#142062=CARTESIAN_POINT ( 'NONE',  ( -12.92414019175886075, 9.417632963106292721, -18.14894846573227127 ) ) ;
#142269=CARTESIAN_POINT ( 'NONE',  ( -12.25000000000000178, 9.349999999999983658, -16.75000000000000000 ) ) ;
#142747=EDGE_LOOP ( 'NONE', ( #15874, #255350, #181976, #32863, #116435 ) ) ;
#142749=VECTOR ( 'NONE', #137757, 1000.000000000000000 ) ;
#142927=CARTESIAN_POINT ( 'NONE',  ( 23.04999999999999716, 8.822561741666397950, -20.84999999999999432 ) ) ;
#142929=EDGE_LOOP ( 'NONE', ( #93135, #108735, #93546, #105337 ) ) ;
#142994=VECTOR ( 'NONE', #41692, 1000.000000000000000 ) ;
#143430=ORIENTED_EDGE ( 'NONE', *, *, #29737, .F. ) ;
#143448=DIRECTION ( 'NONE',  ( 0.000000000000000000, -0.000000000000000000, -1.000000000000000000 ) ) ;
#143544=VERTEX_POINT ( 'NONE', #110164 ) ;
#143568=CARTESIAN_POINT ( 'NONE',  ( 20.05000000000002913, 7.250000000000015099, -9.250000000000001776 ) ) ;
#143641=DIRECTION ( 'NONE',  ( 1.000000000000000000, 0.000000000000000000, 0.000000000000000000 ) ) ;
#143958=CARTESIAN_POINT ( 'NONE',  ( -23.25000000000000355, 11.74999999999998224, -9.250000000000001776 ) ) ;
#143976=CARTESIAN_POINT ( 'NONE',  ( -16.92280123533710068, 9.949999999999983302, -20.64936768591492466 ) ) ;
#144018=VECTOR ( 'NONE', #24387, 1000.000000000000000 ) ;
#144190=ADVANCED_FACE ( 'NONE', ( #219823 ), #98552, .F. ) ;
#144203=DIRECTION ( 'NONE',  ( 0.2834754621636439431, -0.2834754621636535465, -0.9161240771326838450 ) ) ;
#144267=CARTESIAN_POINT ( 'NONE',  ( 20.04999999999999716, 8.750000000000014211, -20.85000000000000142 ) ) ;
#144531=ADVANCED_BREP_SHAPE_REPRESENTATION ( '', ( #105841, #2425 ), #247943 ) ;
#144534=ORIENTED_EDGE ( 'NONE', *, *, #25035, .T. ) ;
#144671=CARTESIAN_POINT ( 'NONE',  ( 18.39999999999999503, 11.74999999999998224, -24.25000000000001066 ) ) ;
#145120=ORIENTED_EDGE ( 'NONE', *, *, #164728, .F. ) ;
#145287=CARTESIAN_POINT ( 'NONE',  ( -18.38817693311004575, 11.48149151589976924, -24.25000000000000000 ) ) ;
#145436=ORIENTED_EDGE ( 'NONE', *, *, #109712, .F. ) ;
#145457=VECTOR ( 'NONE', #245977, 1000.000000000000000 ) ;
#145577=CARTESIAN_POINT ( 'NONE',  ( 23.24999999999999645, 11.74999999999998224, -9.250000000000001776 ) ) ;
#145665=ORIENTED_EDGE ( 'NONE', *, *, #245424, .T. ) ;
#145716=CARTESIAN_POINT ( 'NONE',  ( 18.39999999999999503, 5.649999999999983480, -12.65000000000000213 ) ) ;
#145742=CARTESIAN_POINT ( 'NONE',  ( -16.87331047859649757, 9.949999999999983302, -20.85000000000000142 ) ) ;
#145867=ADVANCED_FACE ( 'NONE', ( #89038 ), #23960, .F. ) ;
#145930=CARTESIAN_POINT ( 'NONE',  ( -17.11825945287481332, 10.04999999999998295, -20.85000000000000142 ) ) ;
#146218=VERTEX_POINT ( 'NONE', #245265 ) ;
#146221=B_SPLINE_CURVE_WITH_KNOTS ( 'NONE', 3,
 ( #183431, #243387, #187291, #169032, #223814, #8639, #84260, #49040, #88133, #167736 ),
 .UNSPECIFIED., .F., .F.,
 ( 4, 3, 3, 4 ),
 ( 1.893216038736613966E-15, 3.877043166999528430E-05, 7.336897548476726920E-05, 7.659383120240106035E-05 ),
 .UNSPECIFIED. ) ;
#146281=DIRECTION ( 'NONE',  ( 0.000000000000000000, 0.000000000000000000, 1.000000000000000000 ) ) ;
#146471=EDGE_LOOP ( 'NONE', ( #71231, #205987, #125174, #191217 ) ) ;
#146533=CARTESIAN_POINT ( 'NONE',  ( 15.66039659514496130, 9.360749169915104417, -17.31457014060726962 ) ) ;
#146642=CARTESIAN_POINT ( 'NONE',  ( -16.81744102076748959, 9.949999999999983302, -20.85000000000000142 ) ) ;
#146906=CIRCLE ( 'NONE', #134262, 14.30833333333333890 ) ;
#147078=CARTESIAN_POINT ( 'NONE',  ( 16.87683809663749557, 9.949999999999976197, -20.85000000000000142 ) ) ;
#147105=CARTESIAN_POINT ( 'NONE',  ( 20.27550659511089037, 9.216043722508848290, -20.84999999999999787 ) ) ;
#147141=VECTOR ( 'NONE', #126681, 1000.000000000000000 ) ;
#147206=CARTESIAN_POINT ( 'NONE',  ( -15.75000000000000000, 9.349999999999983658, -16.86426760761610311 ) ) ;
#147276=EDGE_LOOP ( 'NONE', ( #38000, #255070, #102737, #38110, #23835, #172039, #206364, #139724, #49644, #92111, #57067, #226481, #203162, #105000 ) ) ;
#147317=ADVANCED_FACE ( 'NONE', ( #219473 ), #21319, .F. ) ;
#147392=CARTESIAN_POINT ( 'NONE',  ( -21.64999999999999858, 10.04999999999998295, -12.65000000000000213 ) ) ;
#147422=EDGE_CURVE ( 'NONE', #67836, #75919, #118991, .T. ) ;
#147474=FACE_OUTER_BOUND ( 'NONE', #244146, .T. ) ;
#147502=FACE_OUTER_BOUND ( 'NONE', #186976, .T. ) ;
#147843=VECTOR ( 'NONE', #112041, 1000.000000000000000 ) ;
#147955=CARTESIAN_POINT ( 'NONE',  ( -16.79363873026997922, 9.948850229418431113, -20.84615378144547293 ) ) ;
#147980=ORIENTED_EDGE ( 'NONE', *, *, #203527, .F. ) ;
#148148=PLANE ( 'NONE',  #139269 ) ;
#148360=ORIENTED_EDGE ( 'NONE', *, *, #109150, .F. ) ;
#148395=CARTESIAN_POINT ( 'NONE',  ( -23.25000000000000355, 5.649999999999983480, -12.65000000000000213 ) ) ;
#148477=CARTESIAN_POINT ( 'NONE',  ( -16.94309007106719989, 9.992226192569980014, -12.60579128255550607 ) ) ;
#148837=CARTESIAN_POINT ( 'NONE',  ( -17.11825945287482753, 10.04999999999998295, -12.75000000000000178 ) ) ;
#148877=LINE ( 'NONE', #32808, #59828 ) ;
#149146=CARTESIAN_POINT ( 'NONE',  ( -16.84981964351498718, 9.917318234098837948, -12.86960161401949065 ) ) ;
#149148=CARTESIAN_POINT ( 'NONE',  ( 12.33938619321247288, 9.360723793986032604, -17.31392719460670193 ) ) ;
#149157=CARTESIAN_POINT ( 'NONE',  ( 20.73486653747088582, 7.250000000000026645, -9.250000000000001776 ) ) ;
#149326=PRODUCT ( 'Snap Open Cable Crossbars ', 'Snap Open Cable Crossbars ', '', ( #18241 ) ) ;
#149475=CARTESIAN_POINT ( 'NONE',  ( 18.39999999999999503, 11.47316190336248454, -20.85000000000000142 ) ) ;
#149481=ADVANCED_FACE ( 'NONE', ( #59104 ), #115788, .T. ) ;
#149581=ORIENTED_EDGE ( 'NONE', *, *, #132738, .F. ) ;
#149599=LINE ( 'NONE', #229113, #36592 ) ;
#149618=CARTESIAN_POINT ( 'NONE',  ( -20.65000000000000568, 7.249999999999983125, -20.85000000000000142 ) ) ;
#149779=CARTESIAN_POINT ( 'NONE',  ( -16.93440969289731157, 9.995185175813954714, -12.59123418501079605 ) ) ;
#149782=CIRCLE ( 'NONE', #95590, 0.5000000000000004441 ) ;
#149968=VECTOR ( 'NONE', #49281, 1000.000000000000000 ) ;
#150164=LINE ( 'NONE', #124179, #3084 ) ;
#150343=ORIENTED_EDGE ( 'NONE', *, *, #90030, .F. ) ;
#150430=FACE_OUTER_BOUND ( 'NONE', #128562, .T. ) ;
#150620=ORIENTED_EDGE ( 'NONE', *, *, #45508, .F. ) ;
#150799=EDGE_CURVE ( 'NONE', #5409, #33881, #94914, .T. ) ;
#150997=ORIENTED_EDGE ( 'NONE', *, *, #228165, .F. ) ;
#151003=LINE ( 'NONE', #153613, #12859 ) ;
#151048=CARTESIAN_POINT ( 'NONE',  ( -16.93302609847409457, 9.996682520803211958, -12.58638849536254867 ) ) ;
#151050=VECTOR ( 'NONE', #29712, 1000.000000000000000 ) ;
#151210=ORIENTED_EDGE ( 'NONE', *, *, #193056, .F. ) ;
#151393=DIRECTION ( 'NONE',  ( 0.000000000000000000, 0.000000000000000000, -1.000000000000000000 ) ) ;
#151444=EDGE_CURVE ( 'NONE', #188149, #42380, #46784, .T. ) ;
#151725=CARTESIAN_POINT ( 'NONE',  ( -16.79270642812305070, 9.946244216938156413, -12.66106672143717660 ) ) ;
#151832=EDGE_CURVE ( 'NONE', #219433, #140980, #249147, .T. ) ;
#152067=CARTESIAN_POINT ( 'NONE',  ( 15.48841904831874849, 8.561580951681223794, -20.85000000000000497 ) ) ;
#152383=CARTESIAN_POINT ( 'NONE',  ( -16.87036670365549895, 9.989418819301647545, -12.52043988269794639 ) ) ;
#152464=CARTESIAN_POINT ( 'NONE',  ( -21.65000000000000213, 7.249999999999983125, -12.65000000000000213 ) ) ;
#152545=EDGE_CURVE ( 'NONE', #92740, #86390, #89744, .T. ) ;
#152802=VERTEX_POINT ( 'NONE', #114519 ) ;
#152859=ORIENTED_EDGE ( 'NONE', *, *, #175814, .T. ) ;
#153046=CIRCLE ( 'NONE', #186324, 0.09999999999999939493 ) ;
#153257=CARTESIAN_POINT ( 'NONE',  ( 23.04999999999999716, 8.822561741666397950, -9.250000000000001776 ) ) ;
#153319=CARTESIAN_POINT ( 'NONE',  ( -20.65000000000000568, 5.649999999999983480, -20.85000000000000142 ) ) ;
#153491=CARTESIAN_POINT ( 'NONE',  ( -16.93353400591625757, 10.00461239617294140, -20.93268447020540890 ) ) ;
#153513=CARTESIAN_POINT ( 'NONE',  ( 0.000000000000000000, 0.000000000000000000, 0.000000000000000000 ) ) ;
#153547=CARTESIAN_POINT ( 'NONE',  ( -17.11825945287481332, 10.04999999999998295, -20.75000000000000000 ) ) ;
#153613=CARTESIAN_POINT ( 'NONE',  ( 20.27550659511088682, 9.216043722508844738, -9.250000000000001776 ) ) ;
#153660=B_SPLINE_CURVE_WITH_KNOTS ( 'NONE', 3,
 ( #55278, #134823, #175300, #157008, #216941, #257308, #254751, #38335, #154456, #155735 ),
 .UNSPECIFIED., .F., .F.,
 ( 4, 3, 3, 4 ),
 ( 0.000000000000000000, 4.874959354402336225E-05, 9.785140065120830446E-05, 0.0001360444631935979931 ),
 .UNSPECIFIED. ) ;
#154311=CARTESIAN_POINT ( 'NONE',  ( -16.89935556175729658, 9.949999999999981526, -13.13967636288533036 ) ) ;
#154331=CARTESIAN_POINT ( 'NONE',  ( -17.11825945287481332, 9.949999999999983302, -20.75000000000000000 ) ) ;
#154456=CARTESIAN_POINT ( 'NONE',  ( -16.88495309932522304, 9.954627058472855339, -12.63454867381191526 ) ) ;
#154529=CARTESIAN_POINT ( 'NONE',  ( 14.45204356427542081, 9.450668889167527453, -15.05554649020734814 ) ) ;
#154535=CARTESIAN_POINT ( 'NONE',  ( -16.27683809663750480, 9.349999999999978328, -9.250000000000001776 ) ) ;
#154575=CARTESIAN_POINT ( 'NONE',  ( -18.34374000495060386, 11.47316190336247033, -9.249999999999998224 ) ) ;
#154744=CARTESIAN_POINT ( 'NONE',  ( -16.94107738177414291, 10.01423928513661998, -20.94999999999999929 ) ) ;
#154768=ADVANCED_FACE ( 'NONE', ( #133647 ), #213176, .F. ) ;
#155232=LINE ( 'NONE', #237307, #28535 ) ;
#155323=ORIENTED_EDGE ( 'NONE', *, *, #203527, .T. ) ;
#155478=DIRECTION ( 'NONE',  ( -1.000000000000000000, 0.000000000000000000, 0.000000000000000000 ) ) ;
#155687=CARTESIAN_POINT ( 'NONE',  ( -21.65000000000000213, 9.949999999999985079, -12.75000000000000178 ) ) ;
#155735=CARTESIAN_POINT ( 'NONE',  ( -16.89268316805466341, 9.951721813242185632, -12.64424752145445296 ) ) ;
#155817=ORIENTED_EDGE ( 'NONE', *, *, #102853, .F. ) ;
#155876=CARTESIAN_POINT ( 'NONE',  ( -16.77779411503079032, 9.946101446924121348, -12.66305741761983406 ) ) ;
#156119=CARTESIAN_POINT ( 'NONE',  ( -16.87683809663752399, 9.849999999999988987, -20.09763598180369826 ) ) ;
#156236=CARTESIAN_POINT ( 'NONE',  ( -15.75000000000000355, 9.349999999999983658, -16.75000000000000355 ) ) ;
#156336=AXIS2_PLACEMENT_3D ( 'NONE', #29249, #10937, #9635 ) ;
#156497=CARTESIAN_POINT ( 'NONE',  ( 23.24999999999999645, 11.74999999999998224, -20.84999999999999432 ) ) ;
#156577=PLANE ( 'NONE',  #100450 ) ;
#156963=DIRECTION ( 'NONE',  ( -1.020425574104004196E-15, -1.210927747993693964E-31, 1.000000000000000000 ) ) ;
#157008=CARTESIAN_POINT ( 'NONE',  ( -16.86379686415369861, 9.975217759253158789, -12.56661011090972124 ) ) ;
#157013=CARTESIAN_POINT ( 'NONE',  ( 18.39999999999999503, 11.74999999999998224, -12.65000000000000213 ) ) ;
#157028=CARTESIAN_POINT ( 'NONE',  ( -16.87331047859649757, 9.949999999999983302, -20.85000000000000142 ) ) ;
#157080=DIRECTION ( 'NONE',  ( 0.7071067811865493491, 0.7071067811865456854, 0.000000000000000000 ) ) ;
#157211=PLANE ( 'NONE',  #103278 ) ;
#157284=ORIENTED_EDGE ( 'NONE', *, *, #76450, .F. ) ;
#157349=VECTOR ( 'NONE', #102040, 1000.000000000000000 ) ;
#157453=DIRECTION ( 'NONE',  ( 0.000000000000000000, 0.000000000000000000, -1.000000000000000000 ) ) ;
#157664=EDGE_LOOP ( 'NONE', ( #35911, #73895, #102084, #245067, #189926, #25802 ) ) ;
#157680=ORIENTED_EDGE ( 'NONE', *, *, #105908, .T. ) ;
#157991=ORIENTED_EDGE ( 'NONE', *, *, #109456, .T. ) ;
#158155=CARTESIAN_POINT ( 'NONE',  ( 23.24999999999999645, 8.822561741666397950, -20.84999999999999432 ) ) ;
#158323=CARTESIAN_POINT ( 'NONE',  ( -18.40000000000000213, 11.47316190336248809, -24.25000000000001066 ) ) ;
#158579=VERTEX_POINT ( 'NONE', #58471 ) ;
#159207=EDGE_CURVE ( 'NONE', #43971, #12920, #228831, .T. ) ;
#159260=EDGE_CURVE ( 'NONE', #190837, #226215, #153660, .T. ) ;
#159576=PRESENTATION_STYLE_ASSIGNMENT (( #218232 ) ) ;
#159722=ORIENTED_EDGE ( 'NONE', *, *, #151444, .F. ) ;
#160041=CARTESIAN_POINT ( 'NONE',  ( 23.24999999999999645, 5.649999999999983480, -12.65000000000000746 ) ) ;
#160386=CARTESIAN_POINT ( 'NONE',  ( -14.11361717019516426, 9.457426452488903124, -18.50004186840003939 ) ) ;
#160559=LINE ( 'NONE', #21051, #69674 ) ;
#160698=ORIENTED_EDGE ( 'NONE', *, *, #79249, .F. ) ;
#160995=CARTESIAN_POINT ( 'NONE',  ( -16.83233564386403813, 9.930221796584607574, -20.72452066347563004 ) ) ;
#161201=CARTESIAN_POINT ( 'NONE',  ( -18.40000000000000213, 8.822561741666397950, -9.250000000000001776 ) ) ;
#161255=CARTESIAN_POINT ( 'NONE',  ( -16.85718274719414467, 9.976142314621760931, -12.56334633218240349 ) ) ;
#161256=EDGE_LOOP ( 'NONE', ( #87166, #35502, #31003, #192486 ) ) ;
#161665=CARTESIAN_POINT ( 'NONE',  ( -14.22969084473441725, 9.456007326069306274, -18.48863349414676094 ) ) ;
#161864=CARTESIAN_POINT ( 'NONE',  ( -15.75000000000000355, 9.349999999999983658, -16.75000000000000355 ) ) ;
#161971=B_SPLINE_CURVE_WITH_KNOTS ( 'NONE', 3,
 ( #61888, #119296, #240522, #58005, #102252, #60583, #181834, #76293, #237943, #215799, #155876, #197532, #218365 ),
 .UNSPECIFIED., .F., .F.,
 ( 4, 3, 3, 3, 4 ),
 ( 1.084999851846394431E-16, 1.946463881814436062E-05, 3.922356109943672979E-05, 4.215060953238128886E-05, 4.415117091092174526E-05 ),
 .UNSPECIFIED. ) ;
#162054=LINE ( 'NONE', #65492, #138833 ) ;
#162093=DIRECTION ( 'NONE',  ( 1.000000000000000000, 0.000000000000000000, 0.000000000000000000 ) ) ;
#162294=CARTESIAN_POINT ( 'NONE',  ( -16.78493211734303259, 9.945835743204170853, -20.83605098089596908 ) ) ;
#162464=DIRECTION ( 'NONE',  ( -1.000000000000000000, 0.000000000000000000, 3.469446951953635015E-14 ) ) ;
#162526=CYLINDRICAL_SURFACE ( 'NONE', #116530, 0.5000000000000004441 ) ;
#162752=CARTESIAN_POINT ( 'NONE',  ( -16.92570016628983964, 9.958788957739857395, -20.87934932996099846 ) ) ;
#162787=LINE ( 'NONE', #47942, #61746 ) ;
#162836=CARTESIAN_POINT ( 'NONE',  ( -23.25000000000000355, 10.04999999999998295, -12.75000000000000178 ) ) ;
#162907=( BOUNDED_SURFACE ( )  B_SPLINE_SURFACE ( 3, 2, ( 
 ( #177434, #256882, #78283 ),
 ( #219077, #58709, #138249 ),
 ( #36, #77008, #19621 ),
 ( #120028, #217784, #99122 ) ),
 .UNSPECIFIED., .F., .F., .F. ) 
 B_SPLINE_SURFACE_WITH_KNOTS ( ( 4, 4 ),
 ( 3, 3 ),
 ( 5.727910411845712702, 5.983100554402348337 ),
 ( 0.000000000000000000, 1.000000000000000000 ),
 .UNSPECIFIED. ) 
 GEOMETRIC_REPRESENTATION_ITEM ( )  RATIONAL_B_SPLINE_SURFACE ( (
 ( 1.000000000000000000, 0.8946697475932152699, 1.000000000000000000),
 ( 1.000000000000000000, 0.9035312726220557922, 1.000000000000000000),
 ( 1.000000000000000000, 0.9104333467450282935, 1.000000000000000000),
 ( 1.000000000000000000, 0.9152888060719359675, 1.000000000000000000) ) ) 
 REPRESENTATION_ITEM ( '' )  SURFACE ( )  );
#163025=EDGE_CURVE ( 'NONE', #158579, #190837, #248159, .T. ) ;
#163267=VERTEX_POINT ( 'NONE', #212035 ) ;
#163323=EDGE_CURVE ( 'NONE', #18030, #96167, #232891, .T. ) ;
#163557=CARTESIAN_POINT ( 'NONE',  ( 13.77030915526558275, 9.456007326069306274, -18.48863349414675383 ) ) ;
#163558=CARTESIAN_POINT ( 'NONE',  ( -16.96982749440706328, 9.949999999999983302, -20.37522159118827858 ) ) ;
#163690=ORIENTED_EDGE ( 'NONE', *, *, #235623, .F. ) ;
#163902=VECTOR ( 'NONE', #67881, 1000.000000000000000 ) ;
#163957=ORIENTED_EDGE ( 'NONE', *, *, #90468, .F. ) ;
#163985=CARTESIAN_POINT ( 'NONE',  ( -16.87383368123029825, 9.949999999999983302, -12.65000000000000213 ) ) ;
#164243=ORIENTED_EDGE ( 'NONE', *, *, #132353, .F. ) ;
#164427=LINE ( 'NONE', #143568, #163902 ) ;
#164495=ORIENTED_EDGE ( 'NONE', *, *, #22727, .T. ) ;
#164587=CARTESIAN_POINT ( 'NONE',  ( 18.39999999999997371, 11.47316190336247388, -24.25000000000001066 ) ) ;
#164662=DIRECTION ( 'NONE',  ( -1.000000000000000000, -1.646408749285562691E-14, 1.073024830501117725E-15 ) ) ;
#164712=( LENGTH_UNIT ( ) NAMED_UNIT ( * ) SI_UNIT ( .MILLI., .METRE. ) );
#164728=EDGE_CURVE ( 'NONE', #125620, #184131, #31863, .T. ) ;
#164775=ORIENTED_EDGE ( 'NONE', *, *, #244267, .T. ) ;
#164852=ORIENTED_EDGE ( 'NONE', *, *, #89182, .T. ) ;
#165079=DIRECTION ( 'NONE',  ( 1.186688945009009831E-16, -1.000000000000000000, 0.000000000000000000 ) ) ;
#165124=CARTESIAN_POINT ( 'NONE',  ( -14.00000000000000178, 9.849999999999978328, -16.75000000000000355 ) ) ;
#165479=CARTESIAN_POINT ( 'NONE',  ( -16.93658211146646408, 9.994108662341188776, -12.59570493004432379 ) ) ;
#165557=DIRECTION ( 'NONE',  ( -0.000000000000000000, 0.000000000000000000, -1.000000000000000000 ) ) ;
#166161=CARTESIAN_POINT ( 'NONE',  ( -16.77431908686106610, 9.945805754517978770, -20.83583921765024982 ) ) ;
#166202=VERTEX_POINT ( 'NONE', #168585 ) ;
#166229=EDGE_LOOP ( 'NONE', ( #36403, #65722, #136091, #143430 ) ) ;
#166234=EDGE_LOOP ( 'NONE', ( #194125, #50518, #56132, #82712 ) ) ;
#166266=CARTESIAN_POINT ( 'NONE',  ( -16.77779411440718604, 9.946101447107603022, -20.83694258299546576 ) ) ;
#166311=PLANE ( 'NONE',  #240973 ) ;
#166356=CARTESIAN_POINT ( 'NONE',  ( -18.40000000000000213, 11.47316190336248809, -24.17405393319204876 ) ) ;
#166771=CARTESIAN_POINT ( 'NONE',  ( -21.64999999999999858, 9.349999999999978328, -12.65000000000000213 ) ) ;
#166829=CARTESIAN_POINT ( 'NONE',  ( -16.98495255085917321, 10.00556436599476129, -20.86538279377949578 ) ) ;
#167014=CARTESIAN_POINT ( 'NONE',  ( -15.75000000000000355, 9.349999999999983658, -16.52151937182510366 ) ) ;
#167026=ORIENTED_EDGE ( 'NONE', *, *, #131697, .F. ) ;
#167102=CYLINDRICAL_SURFACE ( 'NONE', #115619, 1.749999999999998002 ) ;
#167296=DIRECTION ( 'NONE',  ( 1.073024830501117725E-15, 0.000000000000000000, 1.000000000000000000 ) ) ;
#167383=LINE ( 'NONE', #8294, #249110 ) ;
#167386=EDGE_CURVE ( 'NONE', #152802, #86042, #218576, .T. ) ;
#167433=CARTESIAN_POINT ( 'NONE',  ( -16.77308656112214891, 9.949999999999983302, -20.84980680829769994 ) ) ;
#167510=EDGE_CURVE ( 'NONE', #106852, #163267, #113547, .T. ) ;
#167727=EDGE_CURVE ( 'NONE', #184131, #195135, #104416, .T. ) ;
#167736=CARTESIAN_POINT ( 'NONE',  ( -16.94445028196808778, 9.992063609697733995, -12.60733017841845438 ) ) ;
#167799=ORIENTED_EDGE ( 'NONE', *, *, #45508, .T. ) ;
#167855=VECTOR ( 'NONE', #251187, 1000.000000000000000 ) ;
#167859=LINE ( 'NONE', #49159, #40128 ) ;
#168439=DIRECTION ( 'NONE',  ( -0.000000000000000000, 1.000000000000000000, -0.000000000000000000 ) ) ;
#168486=CARTESIAN_POINT ( 'NONE',  ( -14.00000000000000178, 9.849999999999978328, -16.75000000000000355 ) ) ;
#168582=LINE ( 'NONE', #32911, #242126 ) ;
#168583=EDGE_LOOP ( 'NONE', ( #59676, #58573, #75103, #250806, #177171, #202423, #202637, #238352, #233705 ) ) ;
#168585=CARTESIAN_POINT ( 'NONE',  ( -18.40000000000000213, 11.48667500175767131, -24.25000000000000000 ) ) ;
#168742=CARTESIAN_POINT ( 'NONE',  ( -16.87333278164150840, 9.882609784578846757, -13.13316780615338075 ) ) ;
#168747=CARTESIAN_POINT ( 'NONE',  ( 15.57250062127603307, 9.370689921602609829, -17.52646512666105139 ) ) ;
#168821=B_SPLINE_CURVE_WITH_KNOTS ( 'NONE', 3,
 ( #47543, #245773, #166266, #248335, #67128, #209203, #147955, #46266, #104930, #146642 ),
 .UNSPECIFIED., .F., .F.,
 ( 4, 3, 3, 4 ),
 ( -2.000561356212805974E-06, 0.000000000000000000, 1.787822682428821068E-05, 4.206475347090201300E-05 ),
 .UNSPECIFIED. ) ;
#169014=PLANE ( 'NONE',  #130146 ) ;
#169032=CARTESIAN_POINT ( 'NONE',  ( -16.92132318717937522, 9.966070024005926342, -12.62240663035206900 ) ) ;
#169033=EDGE_CURVE ( 'NONE', #241787, #222282, #208603, .T. ) ;
#169168=EDGE_LOOP ( 'NONE', ( #100742, #239337 ) ) ;
#169205=ADVANCED_FACE ( 'NONE', ( #246122 ), #25783, .T. ) ;
#169385=CARTESIAN_POINT ( 'NONE',  ( -15.15564720441981628, 9.410708747047081602, -18.06920840584410826 ) ) ;
#169553=ORIENTED_EDGE ( 'NONE', *, *, #150799, .T. ) ;
#169715=CARTESIAN_POINT ( 'NONE',  ( -16.98495255085919098, 10.00556436599476662, -12.63461720622050599 ) ) ;
#169759=DIRECTION ( 'NONE',  ( 1.186688945009010077E-16, -1.000000000000000000, -0.000000000000000000 ) ) ;
#169762=EDGE_LOOP ( 'NONE', ( #238153, #29931, #107585 ) ) ;
#170023=CARTESIAN_POINT ( 'NONE',  ( 13.54577453029515688, 9.450602096088521975, -18.44389596309666501 ) ) ;
#170078=CARTESIAN_POINT ( 'NONE',  ( -16.97683809663753962, 9.949999999999983302, -20.22847083211057750 ) ) ;
#170400=CARTESIAN_POINT ( 'NONE',  ( -21.65000000000000213, 10.04999999999998295, -20.85000000000000142 ) ) ;
#170443=LINE ( 'NONE', #187399, #167855 ) ;
#170461=CARTESIAN_POINT ( 'NONE',  ( -21.65000000000000213, 9.949999999999985079, -12.65000000000000213 ) ) ;
#170489=CARTESIAN_POINT ( 'NONE',  ( -16.94445028196807002, 9.992063609697737547, -20.89266982158155628 ) ) ;
#170527=DIRECTION ( 'NONE',  ( 0.000000000000000000, -1.000000000000000000, 0.000000000000000000 ) ) ;
#170688=CARTESIAN_POINT ( 'NONE',  ( -17.22361732159832215, 10.34515565860243314, -11.37078452586713517 ) ) ;
#170786=EDGE_CURVE ( 'NONE', #194778, #225349, #176921, .T. ) ;
#170794=CARTESIAN_POINT ( 'NONE',  ( -15.75000000000000355, 9.849999999999978328, -16.75000000000000355 ) ) ;
#170987=LINE ( 'NONE', #229631, #209614 ) ;
#171111=ORIENTED_EDGE ( 'NONE', *, *, #78632, .T. ) ;
#171192=ORIENTED_EDGE ( 'NONE', *, *, #132353, .T. ) ;
#171241=CARTESIAN_POINT ( 'NONE',  ( -16.87242674293849731, 9.949999999999983302, -20.85109024637234754 ) ) ;
#171311=CARTESIAN_POINT ( 'NONE',  ( -16.80070461187906972, 9.950000000000081002, -12.64696382916064366 ) ) ;
#171314=ADVANCED_FACE ( 'NONE', ( #4347 ), #242964, .F. ) ;
#171567=LINE ( 'NONE', #128559, #200553 ) ;
#171799=DIRECTION ( 'NONE',  ( 0.000000000000000000, -0.9553114395362878319, -0.2956011730205167498 ) ) ;
#171986=CARTESIAN_POINT ( 'NONE',  ( 18.54999999999999716, 8.750000000000024869, -9.250000000000001776 ) ) ;
#172001=LINE ( 'NONE', #94977, #30247 ) ;
#172035=VECTOR ( 'NONE', #238824, 1000.000000000000000 ) ;
#172039=ORIENTED_EDGE ( 'NONE', *, *, #44478, .F. ) ;
#172529=CARTESIAN_POINT ( 'NONE',  ( -16.91049119928363709, 9.949999999999985079, -20.88172039319084305 ) ) ;
#172555=DIRECTION ( 'NONE',  ( 1.186688945009009831E-16, -1.000000000000000000, 0.000000000000000000 ) ) ;
#172793=AXIS2_PLACEMENT_3D ( 'NONE', #153257, #211926, #32013 ) ;
#172814=CARTESIAN_POINT ( 'NONE',  ( 20.73486653747088582, 7.250000000000026645, -12.65000000000000568 ) ) ;
#172869=CARTESIAN_POINT ( 'NONE',  ( -18.40000000000000213, 11.48667500175766953, -9.250000000000001776 ) ) ;
#173048=CARTESIAN_POINT ( 'NONE',  ( -16.93433913041102912, 10.00597842152393824, -20.93536542739516548 ) ) ;
#173088=DIRECTION ( 'NONE',  ( 0.000000000000000000, -0.000000000000000000, -1.000000000000000000 ) ) ;
#173198=CARTESIAN_POINT ( 'NONE',  ( -18.40000000000000213, 11.33174054712517886, -20.85000000000000142 ) ) ;
#173208=VECTOR ( 'NONE', #6857, 999.9999999999998863 ) ;
#173261=CARTESIAN_POINT ( 'NONE',  ( -16.83794237512074332, 9.926359221107476927, -12.80354215869896173 ) ) ;
#173875=CARTESIAN_POINT ( 'NONE',  ( -16.97683810757273193, 9.949999999999983302, -13.26357671246047687 ) ) ;
#174568=LINE ( 'NONE', #171986, #223201 ) ;
#174758=DIRECTION ( 'NONE',  ( -1.073024830501117725E-15, 0.000000000000000000, 1.000000000000000000 ) ) ;
#175108=CARTESIAN_POINT ( 'NONE',  ( -16.90987985657661596, 9.957807518179730977, -20.86928708888364170 ) ) ;
#175300=CARTESIAN_POINT ( 'NONE',  ( -16.86337532320262156, 9.979967204224358568, -12.55107553101719198 ) ) ;
#175580=EDGE_CURVE ( 'NONE', #226215, #82768, #146221, .T. ) ;
#175725=DIRECTION ( 'NONE',  ( 0.000000000000000000, -1.000000000000000000, 0.000000000000000000 ) ) ;
#175793=CARTESIAN_POINT ( 'NONE',  ( -16.77683809663752257, 9.945835743204145984, -12.66394901910421034 ) ) ;
#175814=EDGE_CURVE ( 'NONE', #209877, #196735, #161971, .T. ) ;
#175872=LINE ( 'NONE', #152464, #147843 ) ;
#176323=ORIENTED_EDGE ( 'NONE', *, *, #1682, .T. ) ;
#176452=LINE ( 'NONE', #79865, #51555 ) ;
#176473=LINE ( 'NONE', #255930, #56289 ) ;
#176837=CARTESIAN_POINT ( 'NONE',  ( -12.25000000000000178, 9.349999999999983658, -16.75000000000000000 ) ) ;
#176872=ORIENTED_EDGE ( 'NONE', *, *, #231915, .T. ) ;
#176885=ORIENTED_EDGE ( 'NONE', *, *, #67547, .F. ) ;
#176921=LINE ( 'NONE', #80320, #51881 ) ;
#176950=FILL_AREA_STYLE ('',( #137772 ) ) ;
#177044=CARTESIAN_POINT ( 'NONE',  ( -16.87683809663752399, 21.23804903843306491, -12.65000000000000213 ) ) ;
#177112=EDGE_LOOP ( 'NONE', ( #81209, #72714, #45994, #212184 ) ) ;
#177149=CARTESIAN_POINT ( 'NONE',  ( -16.93388492042258875, 9.988541822515902169, -12.59945487681382836 ) ) ;
#177171=ORIENTED_EDGE ( 'NONE', *, *, #116110, .T. ) ;
#177395=VERTEX_POINT ( 'NONE', #196490 ) ;
#177434=CARTESIAN_POINT ( 'NONE',  ( -18.44085059012131822, 11.51401249348379530, -9.259694680878462592 ) ) ;
#177509=ORIENTED_EDGE ( 'NONE', *, *, #178791, .T. ) ;
#177546=CARTESIAN_POINT ( 'NONE',  ( -18.40000000000000213, 5.649999999999983480, -20.85000000000000142 ) ) ;
#177601=CARTESIAN_POINT ( 'NONE',  ( 20.05000000000002913, 7.250000000000015099, -12.65000000000000391 ) ) ;
#177842=VECTOR ( 'NONE', #16220, 1000.000000000000000 ) ;
#177995=ADVANCED_FACE ( 'NONE', ( #109917 ), #184941, .T. ) ;
#178432=CARTESIAN_POINT ( 'NONE',  ( -16.87242674293850797, 9.949999999999983302, -12.64890975362765424 ) ) ;
#178564=ADVANCED_FACE ( 'NONE', ( #20491 ), #183405, .F. ) ;
#178791=EDGE_CURVE ( 'NONE', #152802, #158579, #225549, .T. ) ;
#178892=CYLINDRICAL_SURFACE ( 'NONE', #98684, 0.9000000000000014655 ) ;
#178947=DIRECTION ( 'NONE',  ( 1.000000000000000000, -0.000000000000000000, -0.000000000000000000 ) ) ;
#178990=CARTESIAN_POINT ( 'NONE',  ( 20.05000000000002913, 7.250000000000015099, -20.85000000000000142 ) ) ;
#179106=DIRECTION ( 'NONE',  ( 1.186688945009010077E-16, -1.000000000000000000, -0.000000000000000000 ) ) ;
#179128=ORIENTED_EDGE ( 'NONE', *, *, #141580, .F. ) ;
#179287=ORIENTED_EDGE ( 'NONE', *, *, #244879, .F. ) ;
#179288=EDGE_CURVE ( 'NONE', #214183, #88756, #124157, .T. ) ;
#179351=CARTESIAN_POINT ( 'NONE',  ( 18.39999999999999503, 11.74999999999998224, -24.25000000000001066 ) ) ;
#179454=EDGE_LOOP ( 'NONE', ( #197739, #11464, #36004 ) ) ;
#179457=EDGE_CURVE ( 'NONE', #241787, #71101, #32597, .T. ) ;
#179541=CARTESIAN_POINT ( 'NONE',  ( -16.92778301347286884, 10.00094491683533526, -12.57148189203151034 ) ) ;
#180090=EDGE_CURVE ( 'NONE', #258053, #88402, #78925, .T. ) ;
#180100=EDGE_CURVE ( 'NONE', #18030, #68437, #61758, .T. ) ;
#180557=CARTESIAN_POINT ( 'NONE',  ( -16.84981964351497652, 9.917318234098841501, -20.63039838598054843 ) ) ;
#180793=DIRECTION ( 'NONE',  ( -0.000000000000000000, -0.000000000000000000, -1.000000000000000000 ) ) ;
#180813=CARTESIAN_POINT ( 'NONE',  ( -16.91256925476571382, 9.985731158128174911, -12.53235751099473205 ) ) ;
#181107=LINE ( 'NONE', #186230, #41951 ) ;
#181146=VECTOR ( 'NONE', #222926, 1000.000000000000000 ) ;
#181192=LINE ( 'NONE', #82033, #197182 ) ;
#181304=LINE ( 'NONE', #2634, #122566 ) ;
#181378=VERTEX_POINT ( 'NONE', #210314 ) ;
#181424=CARTESIAN_POINT ( 'NONE',  ( -12.29659703204452015, 9.355888454502544249, -16.28864289677800059 ) ) ;
#181618=LINE ( 'NONE', #23843, #157349 ) ;
#181625=PLANE ( 'NONE',  #255457 ) ;
#181809=ORIENTED_EDGE ( 'NONE', *, *, #191807, .T. ) ;
#181834=CARTESIAN_POINT ( 'NONE',  ( -16.78055652883087134, 9.946776916125346091, -12.66079183759242888 ) ) ;
#181836=CARTESIAN_POINT ( 'NONE',  ( -16.87998658237741623, 9.949999999999983302, -20.63636043226203753 ) ) ;
#181962=ORIENTED_EDGE ( 'NONE', *, *, #183428, .T. ) ;
#181976=ORIENTED_EDGE ( 'NONE', *, *, #126436, .T. ) ;
#182119=CARTESIAN_POINT ( 'NONE',  ( -16.97683809663752186, 9.849999999999985434, -12.65000000000000213 ) ) ;
#182377=EDGE_CURVE ( 'NONE', #206683, #116233, #82978, .T. ) ;
#182417=ADVANCED_FACE ( 'NONE', ( #880 ), #84240, .F. ) ;
#182456=ADVANCED_FACE ( 'NONE', ( #6030 ), #124718, .F. ) ;
#182528=DIRECTION ( 'NONE',  ( -0.8049926720990042694, -0.5932847527679310229, 0.000000000000000000 ) ) ;
#182704=CARTESIAN_POINT ( 'NONE',  ( -12.93407622233967658, 9.417789466952205757, -15.35738454397687214 ) ) ;
#182832=CARTESIAN_POINT ( 'NONE',  ( 20.09999999999999787, 9.749999999999982236, -9.250000000000001776 ) ) ;
#182872=EDGE_CURVE ( 'NONE', #254638, #143544, #43590, .T. ) ;
#183117=ADVANCED_FACE ( 'NONE', ( #45525, #101603, #27284 ), #225421, .T. ) ;
#183132=CARTESIAN_POINT ( 'NONE',  ( -16.85697194749130645, 9.908543714123666746, -20.56499573238607326 ) ) ;
#183229=ORIENTED_EDGE ( 'NONE', *, *, #122043, .T. ) ;
#183238=LINE ( 'NONE', #4575, #140204 ) ;
#183405=CYLINDRICAL_SURFACE ( 'NONE', #94715, 0.09999999999999939493 ) ;
#183428=EDGE_CURVE ( 'NONE', #191176, #163267, #204675, .T. ) ;
#183431=CARTESIAN_POINT ( 'NONE',  ( -16.89268316805466341, 9.951721813242185632, -12.64424752145445296 ) ) ;
#183470=ORIENTED_EDGE ( 'NONE', *, *, #71525, .T. ) ;
#183987=CARTESIAN_POINT ( 'NONE',  ( -18.37013991200266005, 11.49974761621197494, -24.29302301051712121 ) ) ;
#184131=VERTEX_POINT ( 'NONE', #255369 ) ;
#184595=DIRECTION ( 'NONE',  ( 0.000000000000000000, 1.000000000000000000, 0.000000000000000000 ) ) ;
#184813=CARTESIAN_POINT ( 'NONE',  ( -16.88219499860498374, 9.950206425427586154, -12.64930969010730699 ) ) ;
#184941=( BOUNDED_SURFACE ( )  B_SPLINE_SURFACE ( 3, 2, ( 
 ( #171241, #172529, #249460 ),
 ( #69540, #211608, #229884 ),
 ( #49948, #134604, #33016 ),
 ( #133354, #210329, #129502 ) ),
 .UNSPECIFIED., .F., .F., .F. ) 
 B_SPLINE_SURFACE_WITH_KNOTS ( ( 4, 4 ),
 ( 3, 3 ),
 ( 3.658908243880901523, 4.712388980384689674 ),
 ( 0.000000000000000000, 1.000000000000000000 ),
 .UNSPECIFIED. ) 
 GEOMETRIC_REPRESENTATION_ITEM ( )  RATIONAL_B_SPLINE_SURFACE ( (
 ( 1.000000000000000000, 0.8984936768950576580, 1.000000000000000000),
 ( 1.000000000000000000, 0.8646876308615482065, 1.000000000000000000),
 ( 1.000000000000000000, 0.7953136715913182719, 1.000000000000000000),
 ( 1.000000000000000000, 0.7071067811865414665, 1.000000000000000000) ) ) 
 REPRESENTATION_ITEM ( '' )  SURFACE ( )  );
#185048=CARTESIAN_POINT ( 'NONE',  ( -12.48127053791144903, 9.376580978043939751, -17.62694624701194002 ) ) ;
#185090=ORIENTED_EDGE ( 'NONE', *, *, #114198, .T. ) ;
#185101=EDGE_LOOP ( 'NONE', ( #87671, #42235 ) ) ;
#185262=VECTOR ( 'NONE', #211734, 1000.000000000000000 ) ;
#186100=DIRECTION ( 'NONE',  ( -0.000000000000000000, 0.000000000000000000, -1.000000000000000000 ) ) ;
#186230=CARTESIAN_POINT ( 'NONE',  ( -18.40000000000000213, 5.649999999999983480, -20.85000000000000142 ) ) ;
#186322=CARTESIAN_POINT ( 'NONE',  ( -16.94445028196808778, 9.992063609697733995, -12.60733017841845438 ) ) ;
#186324=AXIS2_PLACEMENT_3D ( 'NONE', #148837, #25053, #8041 ) ;
#186349=CARTESIAN_POINT ( 'NONE',  ( -15.75000000000000355, 9.349999999999983658, -16.75000000000000355 ) ) ;
#186510=AXIS2_PLACEMENT_3D ( 'NONE', #48122, #182528, #85937 ) ;
#186660=CIRCLE ( 'NONE', #228347, 1.749999999999999778 ) ;
#186721=PLANE ( 'NONE',  #107156 ) ;
#186769=EDGE_CURVE ( 'NONE', #106685, #258053, #193965, .T. ) ;
#186976=EDGE_LOOP ( 'NONE', ( #133964, #203461, #238718, #160698 ) ) ;
#186982=AXIS2_PLACEMENT_3D ( 'NONE', #56522, #53981, #156963 ) ;
#186998=ORIENTED_EDGE ( 'NONE', *, *, #1682, .F. ) ;
#187043=CARTESIAN_POINT ( 'NONE',  ( -18.40000000000000213, 8.822561741666397950, -24.25000000000000000 ) ) ;
#187291=CARTESIAN_POINT ( 'NONE',  ( -16.91247567987037570, 9.959082683669246094, -12.62872445853733616 ) ) ;
#187399=CARTESIAN_POINT ( 'NONE',  ( 21.13736287352038445, 8.046642376383999817, -9.250000000000001776 ) ) ;
#187424=VERTEX_POINT ( 'NONE', #16028 ) ;
#187640=CARTESIAN_POINT ( 'NONE',  ( -15.66061380678753245, 9.360723793986032604, -17.31392719460671970 ) ) ;
#187723=CARTESIAN_POINT ( 'NONE',  ( -18.39999999999999858, 11.47867409999928157, -9.274693216340661905 ) ) ;
#188004=EDGE_CURVE ( 'NONE', #47344, #249899, #219119, .T. ) ;
#188149=VERTEX_POINT ( 'NONE', #245972 ) ;
#188274=PLANE ( 'NONE',  #156336 ) ;
#188355=( BOUNDED_CURVE ( )  B_SPLINE_CURVE ( 3, ( #136348, #37305, #236752, #55522 ),
 .UNSPECIFIED., .F., .T. ) 
 B_SPLINE_CURVE_WITH_KNOTS ( ( 4, 4 ),
 ( 2.589852378279006384, 2.850972632318390154 ),
 .UNSPECIFIED. ) 
 CURVE ( )  GEOMETRIC_REPRESENTATION_ITEM ( )  RATIONAL_B_SPLINE_CURVE ( ( 1.000000000000000000, 0.9943260843901262636, 0.9943260843901262636, 1.000000000000000000 ) ) 
 REPRESENTATION_ITEM ( '' )  );
#188654=CARTESIAN_POINT ( 'NONE',  ( -17.71734398241074260, 10.84235722846456440, -23.22513825300560697 ) ) ;
#189239=CARTESIAN_POINT ( 'NONE',  ( 18.39999999999999503, 5.649999999999983480, -20.85000000000000142 ) ) ;
#189280=FACE_OUTER_BOUND ( 'NONE', #247758, .T. ) ;
#189497=LINE ( 'NONE', #48681, #85983 ) ;
#189763=DIRECTION ( 'NONE',  ( -1.652117596168391700E-15, -1.000000000000000000, 0.000000000000000000 ) ) ;
#189871=EDGE_CURVE ( 'NONE', #18030, #116233, #110286, .T. ) ;
#189926=ORIENTED_EDGE ( 'NONE', *, *, #198586, .T. ) ;
#190087=LINE ( 'NONE', #148395, #149968 ) ;
#190088=ORIENTED_EDGE ( 'NONE', *, *, #235919, .T. ) ;
#190199=ORIENTED_EDGE ( 'NONE', *, *, #51880, .T. ) ;
#190200=CARTESIAN_POINT ( 'NONE',  ( -15.39126916658603506, 9.389571634546408418, -17.81764071236916536 ) ) ;
#190311=EDGE_LOOP ( 'NONE', ( #186998, #61302, #167799, #254281 ) ) ;
#190479=ORIENTED_EDGE ( 'NONE', *, *, #243391, .T. ) ;
#190588=CYLINDRICAL_SURFACE ( 'NONE', #80602, 1.749999999999999778 ) ;
#190688=DIRECTION ( 'NONE',  ( 0.7071067811865456854, -0.7071067811865493491, -0.000000000000000000 ) ) ;
#190837=VERTEX_POINT ( 'NONE', #227778 ) ;
#190858=CARTESIAN_POINT ( 'NONE',  ( 12.68104795156994768, 9.396533993953923414, -17.90593977917329127 ) ) ;
#191176=VERTEX_POINT ( 'NONE', #21033 ) ;
#191217=ORIENTED_EDGE ( 'NONE', *, *, #37678, .T. ) ;
#191224=LINE ( 'NONE', #170400, #50933 ) ;
#191253=CARTESIAN_POINT ( 'NONE',  ( -17.22361732159831504, 10.34515565860243314, -22.12921547413287371 ) ) ;
#191285=EDGE_CURVE ( 'NONE', #229697, #816, #41880, .T. ) ;
#191389=CIRCLE ( 'NONE', #78893, 0.09999999999999910349 ) ;
#191510=CIRCLE ( 'NONE', #195598, 0.09999999999999961697 ) ;
#191807=EDGE_CURVE ( 'NONE', #83518, #187424, #191389, .T. ) ;
#191834=CARTESIAN_POINT ( 'NONE',  ( -16.94445028196808778, 9.992063609697733995, -12.60733017841845438 ) ) ;
#192126=CARTESIAN_POINT ( 'NONE',  ( -16.77308656112214891, 9.949999999999979750, -12.65019319170230716 ) ) ;
#192227=CARTESIAN_POINT ( 'NONE',  ( -18.40000000000000213, 11.47316190336247388, -12.55000000000000249 ) ) ;
#192336=PLANE ( 'NONE',  #205054 ) ;
#192419=CARTESIAN_POINT ( 'NONE',  ( 23.04999999999999716, 8.822561741666397950, -24.25000000000000000 ) ) ;
#192486=ORIENTED_EDGE ( 'NONE', *, *, #46103, .T. ) ;
#192534=DIRECTION ( 'NONE',  ( 0.000000000000000000, 1.000000000000000000, -0.000000000000000000 ) ) ;
#193056=EDGE_CURVE ( 'NONE', #109071, #106852, #62348, .T. ) ;
#193086=CARTESIAN_POINT ( 'NONE',  ( -16.87331047859651179, 9.949999999999986855, -12.65000000000000213 ) ) ;
#193201=ORIENTED_EDGE ( 'NONE', *, *, #186769, .F. ) ;
#193219=ORIENTED_EDGE ( 'NONE', *, *, #209137, .F. ) ;
#193306=EDGE_LOOP ( 'NONE', ( #19583, #103099, #203983, #239578 ) ) ;
#193353=CARTESIAN_POINT ( 'NONE',  ( -16.94333152882356330, 9.990342011457666871, -20.89203153110148747 ) ) ;
#193649=DIRECTION ( 'NONE',  ( 0.000000000000000000, 0.000000000000000000, 1.000000000000000000 ) ) ;
#193931=( NAMED_UNIT ( * ) SI_UNIT ( $, .STERADIAN. ) SOLID_ANGLE_UNIT ( ) );
#193965=LINE ( 'NONE', #31064, #98615 ) ;
#194069=VERTEX_POINT ( 'NONE', #156497 ) ;
#194073=UNCERTAINTY_MEASURE_WITH_UNIT (LENGTH_MEASURE( 1.000000000000000082E-05 ), #236890, 'distance_accuracy_value', 'NONE');
#194084=CARTESIAN_POINT ( 'NONE',  ( 13.99999999999999822, 9.849999999999981881, -16.74999999999999645 ) ) ;
#194125=ORIENTED_EDGE ( 'NONE', *, *, #169033, .F. ) ;
#194217=EDGE_LOOP ( 'NONE', ( #10621, #48592, #164852, #105691, #107591 ) ) ;
#194510=EDGE_CURVE ( 'NONE', #95294, #86390, #168582, .T. ) ;
#194514=MECHANICAL_DESIGN_GEOMETRIC_PRESENTATION_REPRESENTATION('',(#232112),#86309);
#194778=VERTEX_POINT ( 'NONE', #256441 ) ;
#194883=ORIENTED_EDGE ( 'NONE', *, *, #109456, .F. ) ;
#194922=CARTESIAN_POINT ( 'NONE',  ( 12.24999999999999822, 9.349999999999983658, -16.52151937182509656 ) ) ;
#195084=DIRECTION ( 'NONE',  ( -1.000000000000000000, 0.000000000000000000, 0.000000000000000000 ) ) ;
#195093=AXIS2_PLACEMENT_3D ( 'NONE', #14735, #117657, #235048 ) ;
#195135=VERTEX_POINT ( 'NONE', #89418 ) ;
#195162=CARTESIAN_POINT ( 'NONE',  ( -16.93344882324368683, 9.996588767287876820, -20.91302569480492579 ) ) ;
#195203=VERTEX_POINT ( 'NONE', #57982 ) ;
#195204=LINE ( 'NONE', #34847, #43595 ) ;
#195232=SURFACE_STYLE_USAGE ( .BOTH. , #74010 ) ;
#195424=CARTESIAN_POINT ( 'NONE',  ( -16.95709691156388033, 9.949999999999983302, -12.66005756251007774 ) ) ;
#195598=AXIS2_PLACEMENT_3D ( 'NONE', #24301, #144203, #88069 ) ;
#195667=CARTESIAN_POINT ( 'NONE',  ( -17.01473183483382101, 9.949999999999983302, -12.75000000000000178 ) ) ;
#196170=ADVANCED_FACE ( 'NONE', ( #8647 ), #201709, .F. ) ;
#196184=CARTESIAN_POINT ( 'NONE',  ( 14.11444803880196552, 9.457431528848912805, -14.99991693789965730 ) ) ;
#196205=FACE_OUTER_BOUND ( 'NONE', #146471, .T. ) ;
#196295=DIRECTION ( 'NONE',  ( -1.000000000000000000, 0.000000000000000000, 0.000000000000000000 ) ) ;
#196490=CARTESIAN_POINT ( 'NONE',  ( -18.39999999999999858, 11.47316190336247388, -9.325946066807970780 ) ) ;
#196592=CARTESIAN_POINT ( 'NONE',  ( -15.55912972643740488, 8.490870273562565629, -20.94999999999999929 ) ) ;
#196698=CARTESIAN_POINT ( 'NONE',  ( -21.65000000000000213, 7.249999999999983125, -9.250000000000001776 ) ) ;
#196735=VERTEX_POINT ( 'NONE', #74784 ) ;
#196737=VERTEX_POINT ( 'NONE', #154331 ) ;
#196931=ORIENTED_EDGE ( 'NONE', *, *, #94860, .T. ) ;
#197050=DIRECTION ( 'NONE',  ( 0.000000000000000000, 0.000000000000000000, 1.000000000000000000 ) ) ;
#197173=CARTESIAN_POINT ( 'NONE',  ( -16.94389599337535657, 9.991197989756724240, -20.89235519820161358 ) ) ;
#197182=VECTOR ( 'NONE', #256797, 1000.000000000000000 ) ;
#197356=AXIS2_PLACEMENT_3D ( 'NONE', #34413, #253418, #74830 ) ;
#197408=CARTESIAN_POINT ( 'NONE',  ( -16.89081410710458542, 9.951318529847110739, -20.85440591983636693 ) ) ;
#197458=CARTESIAN_POINT ( 'NONE',  ( 15.75000000000000711, 9.349999999999985434, -16.51856895740264619 ) ) ;
#197532=CARTESIAN_POINT ( 'NONE',  ( -16.77732147278574715, 9.945966932573432118, -12.66350875687580846 ) ) ;
#197538=CARTESIAN_POINT ( 'NONE',  ( -16.83199318825828783, 9.930646127981159310, -20.72758518820919704 ) ) ;
#197739=ORIENTED_EDGE ( 'NONE', *, *, #163323, .F. ) ;
#197789=ORIENTED_EDGE ( 'NONE', *, *, #151832, .F. ) ;
#198013=ORIENTED_EDGE ( 'NONE', *, *, #169033, .T. ) ;
#198208=CARTESIAN_POINT ( 'NONE',  ( -16.84421487269768392, 9.949999999999981526, -12.66950212244496043 ) ) ;
#198414=CARTESIAN_POINT ( 'NONE',  ( -17.22767730082269466, 10.34924421246736692, -22.14242869057048324 ) ) ;
#198586=EDGE_CURVE ( 'NONE', #223695, #229697, #247550, .T. ) ;
#198828=CARTESIAN_POINT ( 'NONE',  ( -16.87683809663752399, 9.849999999999988987, -20.09763598180369826 ) ) ;
#199116=DIRECTION ( 'NONE',  ( 1.000000000000000000, -0.000000000000000000, -0.000000000000000000 ) ) ;
#199503=CARTESIAN_POINT ( 'NONE',  ( -13.11924609551135390, 9.431689550524099630, -18.27929003223606585 ) ) ;
#199540=VERTEX_POINT ( 'NONE', #49380 ) ;
#199956=DIRECTION ( 'NONE',  ( 1.000000000000000000, 1.186688945009010077E-16, 0.000000000000000000 ) ) ;
#200022=EDGE_CURVE ( 'NONE', #47766, #209877, #225107, .T. ) ;
#200052=ORIENTED_EDGE ( 'NONE', *, *, #57281, .F. ) ;
#200163=LINE ( 'NONE', #201433, #233530 ) ;
#200257=VERTEX_POINT ( 'NONE', #21515 ) ;
#200500=ORIENTED_EDGE ( 'NONE', *, *, #175580, .F. ) ;
#200553=VECTOR ( 'NONE', #47717, 1000.000000000000000 ) ;
#200963=CARTESIAN_POINT ( 'NONE',  ( -13.43673303185029333, 9.446648990628858655, -15.08916329592318029 ) ) ;
#201066=CARTESIAN_POINT ( 'NONE',  ( 20.73486653747088937, 7.750000000000025757, -20.85000000000000142 ) ) ;
#201157=DIRECTION ( 'NONE',  ( 0.000000000000000000, 0.000000000000000000, -1.000000000000000000 ) ) ;
#201433=CARTESIAN_POINT ( 'NONE',  ( -33.72168855820451938, 9.950000000000001066, -12.64999999999994529 ) ) ;
#201562=DIRECTION ( 'NONE',  ( -3.035766082959430717E-14, 0.000000000000000000, -1.000000000000000000 ) ) ;
#201646=CARTESIAN_POINT ( 'NONE',  ( -16.86445178670637546, 9.962211629115978795, -12.60922256188275092 ) ) ;
#201670=VERTEX_POINT ( 'NONE', #65260 ) ;
#201709=PLANE ( 'NONE',  #2076 ) ;
#201814=CARTESIAN_POINT ( 'NONE',  ( -16.87435696428308063, 9.950002462932223679, -12.64999176516656654 ) ) ;
#201824=CARTESIAN_POINT ( 'NONE',  ( 20.09999999999999787, 9.749999999999982236, -20.84999999999999787 ) ) ;
#202002=DIRECTION ( 'NONE',  ( 1.073024830501117725E-15, 0.000000000000000000, 1.000000000000000000 ) ) ;
#202036=DIRECTION ( 'NONE',  ( 1.000000000000000000, -0.000000000000000000, -0.000000000000000000 ) ) ;
#202054=CARTESIAN_POINT ( 'NONE',  ( -14.56336952470180179, 9.446645344695243196, -18.41080645610019673 ) ) ;
#202132=EDGE_CURVE ( 'NONE', #143544, #188149, #162787, .T. ) ;
#202134=DIRECTION ( 'NONE',  ( -0.000000000000000000, -0.000000000000000000, 1.000000000000000000 ) ) ;
#202253=CARTESIAN_POINT ( 'NONE',  ( -15.52965525596987639, 9.375538102048002642, -15.86987588099083446 ) ) ;
#202309=CARTESIAN_POINT ( 'NONE',  ( 23.24999999999999645, 8.822561741666397950, -12.65000000000000746 ) ) ;
#202423=ORIENTED_EDGE ( 'NONE', *, *, #42989, .F. ) ;
#202446=ORIENTED_EDGE ( 'NONE', *, *, #1084, .T. ) ;
#202547=LINE ( 'NONE', #241674, #61397 ) ;
#202593=ORIENTED_EDGE ( 'NONE', *, *, #209137, .T. ) ;
#202637=ORIENTED_EDGE ( 'NONE', *, *, #236403, .F. ) ;
#202679=CARTESIAN_POINT ( 'NONE',  ( -16.79140778683509794, 9.944941598854562415, -20.82973723377078201 ) ) ;
#202698=VECTOR ( 'NONE', #93149, 1000.000000000000000 ) ;
#202792=CARTESIAN_POINT ( 'NONE',  ( 20.99999999999999645, 9.749999999999982236, -20.84999999999999787 ) ) ;
#202920=FACE_OUTER_BOUND ( 'NONE', #36053, .T. ) ;
#202982=ORIENTED_EDGE ( 'NONE', *, *, #152545, .T. ) ;
#202993=CARTESIAN_POINT ( 'NONE',  ( -16.87683809663752399, 9.949999999999986855, -12.65000000000000213 ) ) ;
#203051=ORIENTED_EDGE ( 'NONE', *, *, #152545, .F. ) ;
#203162=ORIENTED_EDGE ( 'NONE', *, *, #127616, .F. ) ;
#203461=ORIENTED_EDGE ( 'NONE', *, *, #21353, .F. ) ;
#203527=EDGE_CURVE ( 'NONE', #190837, #60760, #191510, .T. ) ;
#203977=VERTEX_POINT ( 'NONE', #111211 ) ;
#203983=ORIENTED_EDGE ( 'NONE', *, *, #167510, .F. ) ;
#204584=EDGE_CURVE ( 'NONE', #33881, #199540, #124827, .T. ) ;
#204601=CARTESIAN_POINT ( 'NONE',  ( -12.26136940704872380, 9.351403174141657004, -16.97953043683849117 ) ) ;
#204617=CARTESIAN_POINT ( 'NONE',  ( -16.94445028196807002, 9.992063609697737547, -20.89266982158155628 ) ) ;
#204675=CIRCLE ( 'NONE', #9058, 0.09999999999999939493 ) ;
#204797=CARTESIAN_POINT ( 'NONE',  ( -14.87779219673428699, 9.430633469072795094, -15.23176579482408499 ) ) ;
#204867=VECTOR ( 'NONE', #230032, 1000.000000000000000 ) ;
#205054=AXIS2_PLACEMENT_3D ( 'NONE', #91942, #231474, #189763 ) ;
#205935=CARTESIAN_POINT ( 'NONE',  ( -23.25000000000000355, 11.74999999999998224, -9.250000000000001776 ) ) ;
#205987=ORIENTED_EDGE ( 'NONE', *, *, #71251, .T. ) ;
#206062=EDGE_LOOP ( 'NONE', ( #110332, #244533, #220944, #231091 ) ) ;
#206364=ORIENTED_EDGE ( 'NONE', *, *, #204584, .F. ) ;
#206387=CARTESIAN_POINT ( 'NONE',  ( -17.01473183483380680, 9.949999999999983302, -20.75000000000000000 ) ) ;
#206498=DIRECTION ( 'NONE',  ( -1.073024830501117725E-15, -0.000000000000000000, -1.000000000000000000 ) ) ;
#206590=CARTESIAN_POINT ( 'NONE',  ( 21.72449340488909897, 10.28395627749112151, -20.84999999999999787 ) ) ;
#206617=ORIENTED_EDGE ( 'NONE', *, *, #83123, .T. ) ;
#206683=VERTEX_POINT ( 'NONE', #51288 ) ;
#206775=EDGE_LOOP ( 'NONE', ( #69940, #198013, #140171, #3672 ) ) ;
#206919=VECTOR ( 'NONE', #80182, 1000.000000000000000 ) ;
#207681=CARTESIAN_POINT ( 'NONE',  ( -16.92507428761700083, 9.949999999999983302, -20.78660254037844624 ) ) ;
#207850=CARTESIAN_POINT ( 'NONE',  ( 15.74999999999999289, 9.349999999999985434, -16.86574316727392286 ) ) ;
#207945=CARTESIAN_POINT ( 'NONE',  ( -18.40000000000000213, 11.47316190336247210, -12.60857864376269255 ) ) ;
#208072=VERTEX_POINT ( 'NONE', #179351 ) ;
#208176=ADVANCED_FACE ( 'NONE', ( #88871 ), #190588, .F. ) ;
#208179=( BOUNDED_SURFACE ( )  B_SPLINE_SURFACE ( 3, 2, ( 
 ( #234519, #115867, #235799 ),
 ( #134125, #213679, #35085 ),
 ( #137970, #195424, #38908 ),
 ( #178432, #57144, #177149 ) ),
 .UNSPECIFIED., .F., .F., .T. ) 
 B_SPLINE_SURFACE_WITH_KNOTS ( ( 4, 4 ),
 ( 3, 3 ),
 ( 4.712388980384689674, 5.765869716888459173 ),
 ( 0.000000000000000000, 1.000000000000000000 ),
 .UNSPECIFIED. ) 
 GEOMETRIC_REPRESENTATION_ITEM ( )  RATIONAL_B_SPLINE_SURFACE ( (
 ( 1.000000000000000000, 0.7071067811865475727, 1.000000000000000000),
 ( 1.000000000000000000, 0.7953136715913138310, 1.000000000000000000),
 ( 1.000000000000000000, 0.8646876308615499829, 1.000000000000000000),
 ( 1.000000000000000000, 0.8984936768950558816, 1.000000000000000000) ) ) 
 REPRESENTATION_ITEM ( '' )  SURFACE ( )  );
#208339=LINE ( 'NONE', #27150, #151050 ) ;
#208453=ORIENTED_EDGE ( 'NONE', *, *, #20595, .F. ) ;
#208534=ORIENTED_EDGE ( 'NONE', *, *, #131697, .T. ) ;
#208603=LINE ( 'NONE', #170794, #246974 ) ;
#208885=APPLICATION_CONTEXT ( 'automotive_design' ) ;
#209094=CARTESIAN_POINT ( 'NONE',  ( -16.85697194749127803, 9.908543714123608126, -12.93500426761395872 ) ) ;
#209129=EDGE_CURVE ( 'NONE', #217199, #214190, #111795, .T. ) ;
#209137=EDGE_CURVE ( 'NONE', #86042, #225349, #195204, .T. ) ;
#209141=ORIENTED_EDGE ( 'NONE', *, *, #21353, .T. ) ;
#209203=CARTESIAN_POINT ( 'NONE',  ( -16.78805706634180694, 9.948252493071178648, -20.84415320803185523 ) ) ;
#209346=CARTESIAN_POINT ( 'NONE',  ( 21.72449340488910607, 10.28395627749112151, -9.250000000000001776 ) ) ;
#209517=ORIENTED_EDGE ( 'NONE', *, *, #163025, .F. ) ;
#209563=CARTESIAN_POINT ( 'NONE',  ( -16.93860193097148326, 9.993107767329243885, -20.90013836730685526 ) ) ;
#209614=VECTOR ( 'NONE', #151393, 1000.000000000000000 ) ;
#209641=CARTESIAN_POINT ( 'NONE',  ( -16.87786941232801041, 9.958154714144969333, -20.87718579979400957 ) ) ;
#209779=DIRECTION ( 'NONE',  ( 1.186688945009009831E-16, -1.000000000000000000, 0.000000000000000000 ) ) ;
#209877=VERTEX_POINT ( 'NONE', #126574 ) ;
#210263=CARTESIAN_POINT ( 'NONE',  ( 20.99999999999999645, 9.749999999999982236, -12.65000000000000568 ) ) ;
#210314=CARTESIAN_POINT ( 'NONE',  ( -21.65000000000000213, 7.249999999999984013, -12.65000000000000213 ) ) ;
#210329=CARTESIAN_POINT ( 'NONE',  ( -17.11825945287482043, 9.949999999999983302, -20.84999999999999787 ) ) ;
#210347=DIRECTION ( 'NONE',  ( -1.000000000000000000, 0.000000000000000000, 0.000000000000000000 ) ) ;
#210400=CARTESIAN_POINT ( 'NONE',  ( 12.26145404764308289, 9.351413679101387544, -16.98034356754895668 ) ) ;
#210561=ORIENTED_EDGE ( 'NONE', *, *, #218716, .T. ) ;
#210595=ADVANCED_FACE ( 'NONE', ( #202920 ), #128524, .T. ) ;
#210609=CARTESIAN_POINT ( 'NONE',  ( -20.65000000000000568, 5.649999999999983480, -9.250000000000001776 ) ) ;
#210679=ADVANCED_FACE ( 'NONE', ( #93234 ), #11145, .T. ) ;
#211018=DIRECTION ( 'NONE',  ( -0.5932847527679299127, 0.8049926720990051576, 6.366092712777055223E-16 ) ) ;
#211544=DIRECTION ( 'NONE',  ( -1.073024830501117725E-15, -0.000000000000000000, -1.000000000000000000 ) ) ;
#211557=FACE_OUTER_BOUND ( 'NONE', #194217, .T. ) ;
#211608=CARTESIAN_POINT ( 'NONE',  ( -16.95709691156346466, 9.949999999999770139, -20.83994243748941599 ) ) ;
#211616=LINE ( 'NONE', #252008, #96006 ) ;
#211690=CARTESIAN_POINT ( 'NONE',  ( 12.25000000000000000, 9.349999999999983658, -16.74999999999999645 ) ) ;
#211734=DIRECTION ( 'NONE',  ( -0.000000000000000000, 1.000000000000000000, 0.000000000000000000 ) ) ;
#211926=DIRECTION ( 'NONE',  ( -0.000000000000000000, -0.000000000000000000, -1.000000000000000000 ) ) ;
#211951=ORIENTED_EDGE ( 'NONE', *, *, #200022, .F. ) ;
#212035=CARTESIAN_POINT ( 'NONE',  ( -16.87683809663752399, 9.849999999999988987, -13.40236401819630530 ) ) ;
#212154=ORIENTED_EDGE ( 'NONE', *, *, #238293, .T. ) ;
#212184=ORIENTED_EDGE ( 'NONE', *, *, #164728, .T. ) ;
#212275=ORIENTED_EDGE ( 'NONE', *, *, #70773, .T. ) ;
#212331=AXIS2_PLACEMENT_3D ( 'NONE', #22093, #202002, #123754 ) ;
#212352=PRODUCT_DEFINITION_CONTEXT ( 'detailed design', #2476, 'design' ) ;
#212355=CARTESIAN_POINT ( 'NONE',  ( -16.80100426158790228, 9.943150520396139669, -12.68294575283405479 ) ) ;
#212402=VERTEX_POINT ( 'NONE', #223884 ) ;
#212808=CARTESIAN_POINT ( 'NONE',  ( -18.40000000000000213, 11.74999999999998224, -12.65000000000000213 ) ) ;
#213003=CARTESIAN_POINT ( 'NONE',  ( -16.89021194854740315, 9.949999999999981526, -20.74256813160433666 ) ) ;
#213176=PLANE ( 'NONE',  #96345 ) ;
#213473=VECTOR ( 'NONE', #51569, 1000.000000000000000 ) ;
#213521=DIRECTION ( 'NONE',  ( -0.000000000000000000, -0.000000000000000000, -1.000000000000000000 ) ) ;
#213600=ADVANCED_FACE ( 'NONE', ( #7806 ), #231665, .F. ) ;
#213605=CARTESIAN_POINT ( 'NONE',  ( -16.85312841634287651, 9.913606177320202661, -12.89717313329253479 ) ) ;
#213631=DIRECTION ( 'NONE',  ( -0.000000000000000000, -0.000000000000000000, -1.000000000000000000 ) ) ;
#213675=AXIS2_PLACEMENT_3D ( 'NONE', #63622, #28391, #45343 ) ;
#213679=CARTESIAN_POINT ( 'NONE',  ( -17.05016517656095942, 9.949999999999985079, -12.67269799599932156 ) ) ;
#214106=DIRECTION ( 'NONE',  ( 1.020425574104004196E-15, 1.210927747993693964E-31, -1.000000000000000000 ) ) ;
#214183=VERTEX_POINT ( 'NONE', #94384 ) ;
#214187=CARTESIAN_POINT ( 'NONE',  ( -16.94165728009536664, 9.987869755923775017, -20.89105500851019670 ) ) ;
#214190=VERTEX_POINT ( 'NONE', #231358 ) ;
#214243=CARTESIAN_POINT ( 'NONE',  ( 12.30626653967341078, 9.356790025045880199, -17.20482650861389118 ) ) ;
#214390=LINE ( 'NONE', #157013, #177842 ) ;
#214509=AXIS2_PLACEMENT_3D ( 'NONE', #124846, #186100, #86963 ) ;
#214684=CARTESIAN_POINT ( 'NONE',  ( -16.93234230245721861, 9.998107370547087314, -20.91769028166625688 ) ) ;
#214877=DIRECTION ( 'NONE',  ( -0.7071067811865456854, 0.7071067811865493491, 0.000000000000000000 ) ) ;
#214895=CARTESIAN_POINT ( 'NONE',  ( -16.87683809663753465, 9.864913778538415556, -13.27571563563853907 ) ) ;
#215256=CARTESIAN_POINT ( 'NONE',  ( 18.54999999999999716, 8.750000000000014211, -12.65000000000000213 ) ) ;
#215458=CARTESIAN_POINT ( 'NONE',  ( -16.89268316805465986, 9.951721813242182080, -20.85575247854553993 ) ) ;
#215544=ORIENTED_EDGE ( 'NONE', *, *, #1268, .T. ) ;
#215728=CARTESIAN_POINT ( 'NONE',  ( 13.22261339317536333, 9.436552840004416964, -15.17795547276030632 ) ) ;
#215799=CARTESIAN_POINT ( 'NONE',  ( -16.77828822508139694, 9.946229374920743993, -12.66262825137395254 ) ) ;
#215846=DIRECTION ( 'NONE',  ( 0.000000000000000000, 0.000000000000000000, -1.000000000000000000 ) ) ;
#216489=CARTESIAN_POINT ( 'NONE',  ( -16.90137573187934095, 9.949999999999986855, -12.78841742409689886 ) ) ;
#216553=CARTESIAN_POINT ( 'NONE',  ( -18.40000000000000213, 11.47316190336248809, -24.17405393319204876 ) ) ;
#216772=DIRECTION ( 'NONE',  ( 1.000000000000000000, 0.000000000000000000, 0.000000000000000000 ) ) ;
#216927=ORIENTED_EDGE ( 'NONE', *, *, #72913, .F. ) ;
#216941=CARTESIAN_POINT ( 'NONE',  ( -16.86422026484316916, 9.970447360860653419, -12.58221322567300859 ) ) ;
#216961=CARTESIAN_POINT ( 'NONE',  ( -16.88328101497759448, 9.950352834218858078, -20.85117951492928157 ) ) ;
#217014=CARTESIAN_POINT ( 'NONE',  ( 15.39793903038207290, 9.389686005655649481, -15.67284350635130430 ) ) ;
#217028=CARTESIAN_POINT ( 'NONE',  ( -16.89268316805465986, 9.951721813242182080, -20.85575247854553993 ) ) ;
#217183=FACE_OUTER_BOUND ( 'NONE', #58080, .T. ) ;
#217199=VERTEX_POINT ( 'NONE', #149618 ) ;
#217722=ORIENTED_EDGE ( 'NONE', *, *, #21382, .T. ) ;
#217784=CARTESIAN_POINT ( 'NONE',  ( -16.91256925476570672, 9.985731158128174911, -12.53235751099471962 ) ) ;
#217833=CARTESIAN_POINT ( 'NONE',  ( -21.65000000000000213, 9.949999999999985079, -20.75000000000000000 ) ) ;
#218155=ORIENTED_EDGE ( 'NONE', *, *, #151444, .T. ) ;
#218232=SURFACE_STYLE_USAGE ( .BOTH. , #138680 ) ;
#218365=CARTESIAN_POINT ( 'NONE',  ( -16.77683809663752257, 9.945835743204145984, -12.66394901910421034 ) ) ;
#218576=LINE ( 'NONE', #161201, #142749 ) ;
#218716=EDGE_CURVE ( 'NONE', #140173, #53539, #43813, .T. ) ;
#219008=DIRECTION ( 'NONE',  ( 0.000000000000000000, -1.000000000000000000, 0.000000000000000000 ) ) ;
#219015=CARTESIAN_POINT ( 'NONE',  ( 12.25000000000000000, 9.849999999999981881, -16.74999999999999645 ) ) ;
#219077=CARTESIAN_POINT ( 'NONE',  ( -17.80356949363960339, 10.87673139700207869, -10.28692697577638171 ) ) ;
#219119=CIRCLE ( 'NONE', #110992, 1.500000000000001332 ) ;
#219179=ORIENTED_EDGE ( 'NONE', *, *, #245424, .F. ) ;
#219426=ORIENTED_EDGE ( 'NONE', *, *, #32846, .T. ) ;
#219433=VERTEX_POINT ( 'NONE', #127746 ) ;
#219473=FACE_OUTER_BOUND ( 'NONE', #16728, .T. ) ;
#219661=CARTESIAN_POINT ( 'NONE',  ( -16.97683810757273193, 9.949999999999983302, -20.23642328753963682 ) ) ;
#219669=CARTESIAN_POINT ( 'NONE',  ( -16.87372397896795206, 9.880599536641732072, -20.35072451003573946 ) ) ;
#219811=AXIS2_PLACEMENT_3D ( 'NONE', #210263, #167296, #69473 ) ;
#219823=FACE_OUTER_BOUND ( 'NONE', #84740, .T. ) ;
#220357=CARTESIAN_POINT ( 'NONE',  ( -20.65000000000000568, 5.649999999999983480, -12.65000000000000213 ) ) ;
#220376=DIRECTION ( 'NONE',  ( 1.000000000000000000, 0.000000000000000000, 0.000000000000000000 ) ) ;
#220395=DIRECTION ( 'NONE',  ( -1.000000000000000000, 1.652117596168391700E-15, 0.000000000000000000 ) ) ;
#220537=CARTESIAN_POINT ( 'NONE',  ( -14.77738660682463667, 9.436552840004420517, -15.17795547276031520 ) ) ;
#220649=CARTESIAN_POINT ( 'NONE',  ( 15.74999999999999645, 9.849999999999981881, -16.74999999999999645 ) ) ;
#220811=CARTESIAN_POINT ( 'NONE',  ( -18.39999999999999858, 11.74999999999998224, -9.250000000000001776 ) ) ;
#220826=CARTESIAN_POINT ( 'NONE',  ( -33.72168855820451938, 9.950000000000001066, -20.85000000000005471 ) ) ;
#220942=CARTESIAN_POINT ( 'NONE',  ( -16.82542659449979539, 9.934499891427430285, -20.75536439997388527 ) ) ;
#220944=ORIENTED_EDGE ( 'NONE', *, *, #126436, .F. ) ;
#221060=DIRECTION ( 'NONE',  ( 1.000000000000000000, 0.000000000000000000, -0.000000000000000000 ) ) ;
#221110=AXIS2_PLACEMENT_3D ( 'NONE', #248472, #107668, #71137 ) ;
#221137=EDGE_LOOP ( 'NONE', ( #256304, #145120, #216927, #212275, #34232, #155817, #101325, #159722, #68983, #109459, #77264, #193219 ) ) ;
#221397=CARTESIAN_POINT ( 'NONE',  ( -16.85718274719399545, 9.976142314621760931, -20.93665366781759474 ) ) ;
#221585=CARTESIAN_POINT ( 'NONE',  ( -13.54036565897075306, 9.451541661385510551, -18.45387549883059464 ) ) ;
#221630=ORIENTED_EDGE ( 'NONE', *, *, #167727, .F. ) ;
#221688=EDGE_CURVE ( 'NONE', #208072, #42380, #8359, .T. ) ;
#221802=CARTESIAN_POINT ( 'NONE',  ( -17.27223548803194575, 10.34539739140540604, -22.13360617919591533 ) ) ;
#222084=DIRECTION ( 'NONE',  ( 1.000000000000000000, -0.000000000000000000, -0.000000000000000000 ) ) ;
#222175=VERTEX_POINT ( 'NONE', #231914 ) ;
#222214=CARTESIAN_POINT ( 'NONE',  ( -16.87333278164143735, 9.882609784578759715, -20.36683219384677912 ) ) ;
#222282=VERTEX_POINT ( 'NONE', #156236 ) ;
#222461=CIRCLE ( 'NONE', #197356, 0.9000000000000014655 ) ;
#222926=DIRECTION ( 'NONE',  ( 0.000000000000000000, 0.000000000000000000, 1.000000000000000000 ) ) ;
#223105=CARTESIAN_POINT ( 'NONE',  ( -17.80356949363898877, 10.87673139700146763, -23.21307302422549768 ) ) ;
#223201=VECTOR ( 'NONE', #213631, 1000.000000000000000 ) ;
#223394=CARTESIAN_POINT ( 'NONE',  ( -16.27683809663751191, 9.349999999999978328, -9.249999999999966249 ) ) ;
#223421=AXIS2_PLACEMENT_3D ( 'NONE', #95957, #236749, #137643 ) ;
#223515=CARTESIAN_POINT ( 'NONE',  ( -16.85312964099708921, 9.913604682067711948, -20.60281570643044802 ) ) ;
#223648=EDGE_CURVE ( 'NONE', #194778, #195203, #22712, .T. ) ;
#223695=VERTEX_POINT ( 'NONE', #155687 ) ;
#223770=ADVANCED_FACE ( 'NONE', ( #38280 ), #94382, .F. ) ;
#223814=CARTESIAN_POINT ( 'NONE',  ( -16.92925196614875816, 9.972331796410120575, -12.61674484771679694 ) ) ;
#223822=DIRECTION ( 'NONE',  ( -1.000000000000000000, 0.000000000000000000, 0.000000000000000000 ) ) ;
#223881=ADVANCED_FACE ( 'NONE', ( #40874 ), #413, .F. ) ;
#223884=CARTESIAN_POINT ( 'NONE',  ( -20.65000000000000568, 7.249999999999983125, -12.65000000000000213 ) ) ;
#224371=CARTESIAN_POINT ( 'NONE',  ( -15.15766958671843412, 9.410538608528867144, -15.43268799714089035 ) ) ;
#224919=ORIENTED_EDGE ( 'NONE', *, *, #228165, .T. ) ;
#224939=SHAPE_REPRESENTATION ( 'Snap Open Cable Crossbars ', ( #2425 ), #247943 ) ;
#224942=DIRECTION ( 'NONE',  ( -1.000000000000000000, 0.000000000000000000, -1.020425574104004196E-15 ) ) ;
#224981=CARTESIAN_POINT ( 'NONE',  ( -17.78043020864321022, 10.85359211200569085, -23.16304916572022066 ) ) ;
#225107=LINE ( 'NONE', #202993, #144018 ) ;
#225205=CARTESIAN_POINT ( 'NONE',  ( -16.87487986503753845, 9.950007555085599975, -12.64997473968673347 ) ) ;
#225297=CARTESIAN_POINT ( 'NONE',  ( -17.11825945287482753, 9.949999999999983302, -12.75000000000000178 ) ) ;
#225349=VERTEX_POINT ( 'NONE', #212808 ) ;
#225373=( BOUNDED_CURVE ( )  B_SPLINE_CURVE ( 3, ( #111686, #191253, #188654, #226475 ),
 .UNSPECIFIED., .F., .T. ) 
 B_SPLINE_CURVE_WITH_KNOTS ( ( 4, 4 ),
 ( 0.3000847527772389500, 0.5517402753107891744 ),
 .UNSPECIFIED. ) 
 CURVE ( )  GEOMETRIC_REPRESENTATION_ITEM ( )  RATIONAL_B_SPLINE_CURVE ( ( 1.000000000000000000, 0.9947294176030464508, 0.9947294176030464508, 1.000000000000000000 ) ) 
 REPRESENTATION_ITEM ( '' )  );
#225421=CYLINDRICAL_SURFACE ( 'NONE', #38113, 14.30833333333333890 ) ;
#225549=B_SPLINE_CURVE_WITH_KNOTS ( 'NONE', 3,
 ( #172869, #231523, #252340, #114118, #15047, #94554, #154575 ),
 .UNSPECIFIED., .F., .F.,
 ( 4, 3, 4 ),
 ( 0.000000000000000000, 4.520325912680724513E-05, 5.794988040901477241E-05 ),
 .UNSPECIFIED. ) ;
#226062=CARTESIAN_POINT ( 'NONE',  ( 15.69410316191958898, 9.356746017078247490, -17.20335972136419755 ) ) ;
#226076=EDGE_CURVE ( 'NONE', #86390, #196737, #242788, .T. ) ;
#226215=VERTEX_POINT ( 'NONE', #235585 ) ;
#226475=CARTESIAN_POINT ( 'NONE',  ( -18.34374000495059676, 11.47316190336247388, -24.25000000000001066 ) ) ;
#226481=ORIENTED_EDGE ( 'NONE', *, *, #72913, .T. ) ;
#226528=CARTESIAN_POINT ( 'NONE',  ( -16.89797118371577156, 9.976380722644002219, -20.93729336755886905 ) ) ;
#226823=CARTESIAN_POINT ( 'NONE',  ( -18.40000000000000213, 11.48667500175766953, -9.250000000000001776 ) ) ;
#227411=EDGE_CURVE ( 'NONE', #226215, #47766, #141322, .T. ) ;
#227470=CARTESIAN_POINT ( 'NONE',  ( -18.40000000000000213, 11.33174054712516110, -12.65000000000000213 ) ) ;
#227714=DIRECTION ( 'NONE',  ( 0.7071067811865463515, 0.7071067811865487940, 7.587431340288849180E-16 ) ) ;
#227736=EDGE_LOOP ( 'NONE', ( #208534, #215544, #96109, #202593, #117908, #233518 ) ) ;
#227778=CARTESIAN_POINT ( 'NONE',  ( -16.87036670365549895, 9.989418819301647545, -12.52043988269794639 ) ) ;
#228032=CARTESIAN_POINT ( 'NONE',  ( -15.73854595235691889, 9.351413679101387544, -16.98034356754896734 ) ) ;
#228135=CARTESIAN_POINT ( 'NONE',  ( 18.39999999999999503, 5.649999999999983480, -24.25000000000001066 ) ) ;
#228165=EDGE_CURVE ( 'NONE', #28990, #14615, #12016, .T. ) ;
#228344=ORIENTED_EDGE ( 'NONE', *, *, #235623, .T. ) ;
#228347=AXIS2_PLACEMENT_3D ( 'NONE', #95526, #172555, #73432 ) ;
#228386=AXIS2_PLACEMENT_3D ( 'NONE', #201066, #58955, #216772 ) ;
#228635=B_SPLINE_CURVE_WITH_KNOTS ( 'NONE', 3,
 ( #63181, #85297, #244392, #140145, #145287, #61916, #100984 ),
 .UNSPECIFIED., .F., .F.,
 ( 4, 3, 4 ),
 ( 0.000000000000000000, 3.882884552234470657E-05, 5.798605692158490785E-05 ),
 .UNSPECIFIED. ) ;
#228680=CARTESIAN_POINT ( 'NONE',  ( -16.85722902420156544, 9.949999999999983302, -12.76554747377053545 ) ) ;
#228683=CARTESIAN_POINT ( 'NONE',  ( 12.60873083341396850, 9.389571634546411971, -17.81764071236915825 ) ) ;
#228827=CARTESIAN_POINT ( 'NONE',  ( 18.39999999999999503, 5.649999999999983480, -12.65000000000000213 ) ) ;
#228831=LINE ( 'NONE', #232689, #202698 ) ;
#228836=B_SPLINE_CURVE_WITH_KNOTS ( 'NONE', 3,
 ( #186322, #148477, #248859, #130175, #66368, #88468, #165479, #149779, #151048, #128915, #10255, #244999, #126334, #105453, #89765, #85894, #125067, #110625, #71527 ),
 .UNSPECIFIED., .F., .F.,
 ( 4, 3, 3, 3, 3, 3, 4 ),
 ( 0.0001624081864585773726, 0.0001685232196531712882, 0.0001764526673566857657, 0.0001916878551483174834, 0.0002009890782182555721, 0.0002238845907555098180, 0.0002283406619926331546 ),
 .UNSPECIFIED. ) ;
#229113=CARTESIAN_POINT ( 'NONE',  ( 15.74999999999999645, 9.849999999999981881, -16.74999999999999645 ) ) ;
#229317=EDGE_CURVE ( 'NONE', #196737, #258053, #4390, .T. ) ;
#229327=CARTESIAN_POINT ( 'NONE',  ( -15.57281606413133979, 9.370655051123479851, -17.52582325598087820 ) ) ;
#229631=CARTESIAN_POINT ( 'NONE',  ( -16.87683809663752399, 9.849999999999985434, -12.65000000000000213 ) ) ;
#229633=EDGE_CURVE ( 'NONE', #214190, #67836, #160559, .T. ) ;
#229687=DIRECTION ( 'NONE',  ( -0.000000000000000000, 1.000000000000000000, -0.000000000000000000 ) ) ;
#229697=VERTEX_POINT ( 'NONE', #147392 ) ;
#229884=CARTESIAN_POINT ( 'NONE',  ( -16.97092634996658944, 10.00088896634839664, -20.86985723370230872 ) ) ;
#229942=CARTESIAN_POINT ( 'NONE',  ( -16.88783316861816530, 9.949999999999983302, -12.75226404197977104 ) ) ;
#229961=DIRECTION ( 'NONE',  ( -1.000000000000000000, -0.000000000000000000, -0.000000000000000000 ) ) ;
#230032=DIRECTION ( 'NONE',  ( -1.020425574104004196E-15, 0.000000000000000000, 1.000000000000000000 ) ) ;
#231091=ORIENTED_EDGE ( 'NONE', *, *, #191285, .F. ) ;
#231252=CARTESIAN_POINT ( 'NONE',  ( -16.77180007708460963, 9.949999999999983302, -12.63561411895481790 ) ) ;
#231358=CARTESIAN_POINT ( 'NONE',  ( -21.65000000000000213, 7.249999999999984013, -20.85000000000000142 ) ) ;
#231474=DIRECTION ( 'NONE',  ( -1.000000000000000000, 1.652117596168391700E-15, 0.000000000000000000 ) ) ;
#231523=CARTESIAN_POINT ( 'NONE',  ( -18.38639463286148867, 11.48019957383597855, -9.250000000000001776 ) ) ;
#231530=CIRCLE ( 'NONE', #6649, 0.1999999999999987899 ) ;
#231624=ADVANCED_FACE ( 'NONE', ( #90923 ), #130039, .F. ) ;
#231665=PLANE ( 'NONE',  #11925 ) ;
#231914=CARTESIAN_POINT ( 'NONE',  ( 12.25000000000000000, 9.849999999999981881, -16.74999999999999645 ) ) ;
#231915=EDGE_CURVE ( 'NONE', #43971, #203977, #128445, .T. ) ;
#231917=CARTESIAN_POINT ( 'NONE',  ( -16.81453046979149235, 9.939102281440909792, -12.71172652360302635 ) ) ;
#232112=STYLED_ITEM ( 'NONE', ( #159576 ), #105841 ) ;
#232242=ORIENTED_EDGE ( 'NONE', *, *, #109712, .T. ) ;
#232477=ADVANCED_FACE ( 'NONE', ( #242344 ), #28482, .T. ) ;
#232656=CARTESIAN_POINT ( 'NONE',  ( 13.99999999999999822, 9.849999999999981881, -16.74999999999999645 ) ) ;
#232689=CARTESIAN_POINT ( 'NONE',  ( 23.24999999999999645, 8.822561741666397950, -9.250000000000001776 ) ) ;
#232760=CARTESIAN_POINT ( 'NONE',  ( 13.54556439290364445, 9.450592112133699985, -15.05618831880839181 ) ) ;
#232782=ADVANCED_FACE ( 'NONE', ( #827 ), #162526, .T. ) ;
#232891=LINE ( 'NONE', #152067, #104177 ) ;
#232999=CARTESIAN_POINT ( 'NONE',  ( -16.93211319090181632, 9.999986781157469196, -20.92250549927306835 ) ) ;
#233055=DIRECTION ( 'NONE',  ( -1.000000000000000000, 0.000000000000000000, 0.000000000000000000 ) ) ;
#233518=ORIENTED_EDGE ( 'NONE', *, *, #223648, .T. ) ;
#233530=VECTOR ( 'NONE', #196295, 1000.000000000000000 ) ;
#233632=ORIENTED_EDGE ( 'NONE', *, *, #250444, .T. ) ;
#233705=ORIENTED_EDGE ( 'NONE', *, *, #236971, .F. ) ;
#233760=EDGE_CURVE ( 'NONE', #199540, #7969, #151003, .T. ) ;
#233860=CARTESIAN_POINT ( 'NONE',  ( -16.81744102076748959, 9.949999999999983302, -20.85000000000000142 ) ) ;
#233915=CARTESIAN_POINT ( 'NONE',  ( -18.40000000000000213, 5.649999999999983480, -24.25000000000001066 ) ) ;
#234018=CARTESIAN_POINT ( 'NONE',  ( 15.06592377766032698, 9.417789466952205757, -15.35738454397687036 ) ) ;
#234025=DIRECTION ( 'NONE',  ( 0.000000000000000000, 0.000000000000000000, -1.000000000000000000 ) ) ;
#234286=DIRECTION ( 'NONE',  ( -0.000000000000000000, 1.000000000000000000, -0.000000000000000000 ) ) ;
#234444=( BOUNDED_SURFACE ( )  B_SPLINE_SURFACE ( 3, 2, ( 
 ( #99290, #22370, #237547 ),
 ( #118899, #221802, #198414 ),
 ( #223105, #2765, #43202 ),
 ( #100562, #23666, #183987 ) ),
 .UNSPECIFIED., .F., .F., .F. ) 
 B_SPLINE_SURFACE_WITH_KNOTS ( ( 4, 4 ),
 ( 3, 3 ),
 ( 0.3000847527772379508, 0.5552748953338751958 ),
 ( 0.000000000000000000, 1.000000000000000000 ),
 .UNSPECIFIED. ) 
 GEOMETRIC_REPRESENTATION_ITEM ( )  RATIONAL_B_SPLINE_SURFACE ( (
 ( 1.000000000000000000, 0.9152888060719377439, 1.000000000000000000),
 ( 1.000000000000000000, 0.9104333467450277384, 1.000000000000000000),
 ( 1.000000000000000000, 0.9035312726220520174, 1.000000000000000000),
 ( 1.000000000000000000, 0.8946697475932143817, 1.000000000000000000) ) ) 
 REPRESENTATION_ITEM ( '' )  SURFACE ( )  );
#234499=DIRECTION ( 'NONE',  ( 1.000000000000000000, 1.646408749285562691E-14, 1.073024830501117725E-15 ) ) ;
#234519=CARTESIAN_POINT ( 'NONE',  ( -17.11825945287482753, 9.949999999999983302, -12.75000000000000178 ) ) ;
#234959=EDGE_LOOP ( 'NONE', ( #150620, #95976, #171111, #97942 ) ) ;
#235034=ORIENTED_EDGE ( 'NONE', *, *, #202132, .T. ) ;
#235039=CARTESIAN_POINT ( 'NONE',  ( -16.90128866880176162, 9.953795777202955719, -20.86267618338863983 ) ) ;
#235048=DIRECTION ( 'NONE',  ( 0.000000000000000000, 1.000000000000000000, 0.000000000000000000 ) ) ;
#235585=CARTESIAN_POINT ( 'NONE',  ( -16.89268316805466341, 9.951721813242185632, -12.64424752145445296 ) ) ;
#235623=EDGE_CURVE ( 'NONE', #53539, #68437, #146906, .T. ) ;
#235734=CARTESIAN_POINT ( 'NONE',  ( -16.81930730667006912, 9.936998068874046908, -12.72676773053820476 ) ) ;
#235799=CARTESIAN_POINT ( 'NONE',  ( -17.11825945287482753, 10.04999999999998295, -12.65000000000000391 ) ) ;
#235919=EDGE_CURVE ( 'NONE', #95294, #188149, #172001, .T. ) ;
#235947=B_SPLINE_CURVE_WITH_KNOTS ( 'NONE', 3,
 ( #115084, #197173, #193353, #14727, #214187, #58924, #78506, #16009, #75959, #95513, #175108, #235039, #215458 ),
 .UNSPECIFIED., .F., .F.,
 ( 4, 3, 3, 3, 4 ),
 ( -3.224855718277970714E-06, -8.470329472543003391E-22, 6.199515528667107161E-06, 4.034952380127394394E-05, 7.452715123699289962E-05 ),
 .UNSPECIFIED. ) ;
#236403=EDGE_CURVE ( 'NONE', #50885, #17161, #56794, .T. ) ;
#236530=CARTESIAN_POINT ( 'NONE',  ( -16.87665923198281348, 9.949999999999983302, -20.85000000000000142 ) ) ;
#236577=CARTESIAN_POINT ( 'NONE',  ( 12.84233041328156766, 9.410538608528868920, -15.43268799714089035 ) ) ;
#236749=DIRECTION ( 'NONE',  ( 0.000000000000000000, -1.000000000000000000, 0.000000000000000000 ) ) ;
#236752=CARTESIAN_POINT ( 'NONE',  ( 17.23472005113827876, 10.30788195450076650, -11.45342313993132599 ) ) ;
#236890=( LENGTH_UNIT ( ) NAMED_UNIT ( * ) SI_UNIT ( .MILLI., .METRE. ) );
#236971=EDGE_CURVE ( 'NONE', #181378, #212402, #175872, .T. ) ;
#237173=VERTEX_POINT ( 'NONE', #201824 ) ;
#237290=SHAPE_DEFINITION_REPRESENTATION ( #65914, #224939 ) ;
#237307=CARTESIAN_POINT ( 'NONE',  ( 18.39999999999999503, 8.822561741666397950, -24.25000000000000000 ) ) ;
#237547=CARTESIAN_POINT ( 'NONE',  ( -16.87036670365548474, 9.989418819301642216, -20.97956011730203940 ) ) ;
#237783=DIRECTION ( 'NONE',  ( -1.186688945009010077E-16, 1.000000000000000000, 0.000000000000000000 ) ) ;
#237823=FILL_AREA_STYLE_COLOUR ( '', #244537 ) ;
#237943=CARTESIAN_POINT ( 'NONE',  ( -16.77902162784673479, 9.946419257207841369, -12.66199124406934118 ) ) ;
#237944=CARTESIAN_POINT ( 'NONE',  ( -16.87683809663752044, 9.949999999999983302, -20.09763598180368405 ) ) ;
#237949=CARTESIAN_POINT ( 'NONE',  ( -16.85939681242906119, 9.905225185925303322, -20.53992195519148467 ) ) ;
#238153=ORIENTED_EDGE ( 'NONE', *, *, #105804, .F. ) ;
#238161=( NAMED_UNIT ( * ) PLANE_ANGLE_UNIT ( ) SI_UNIT ( $, .RADIAN. ) );
#238205=AXIS2_PLACEMENT_3D ( 'NONE', #95450, #32958, #112465 ) ;
#238293=EDGE_CURVE ( 'NONE', #86497, #223695, #189497, .T. ) ;
#238352=ORIENTED_EDGE ( 'NONE', *, *, #37678, .F. ) ;
#238398=DIRECTION ( 'NONE',  ( -0.000000000000000000, -0.000000000000000000, -1.000000000000000000 ) ) ;
#238467=CARTESIAN_POINT ( 'NONE',  ( -17.11825945287481332, 10.04999999999998295, -20.85000000000000142 ) ) ;
#238687=CARTESIAN_POINT ( 'NONE',  ( -18.40000000000000213, 11.47867409999990329, -24.22530678365939494 ) ) ;
#238718=ORIENTED_EDGE ( 'NONE', *, *, #16707, .T. ) ;
#238824=DIRECTION ( 'NONE',  ( 0.000000000000000000, -1.000000000000000000, 0.000000000000000000 ) ) ;
#239032=EDGE_LOOP ( 'NONE', ( #81849, #20381, #118017, #203051, #92895 ) ) ;
#239337=ORIENTED_EDGE ( 'NONE', *, *, #101380, .T. ) ;
#239501=CARTESIAN_POINT ( 'NONE',  ( -16.87036670365549895, 9.989418819301645769, -12.52043988269794816 ) ) ;
#239578=ORIENTED_EDGE ( 'NONE', *, *, #67547, .T. ) ;
#239814=( BOUNDED_SURFACE ( )  B_SPLINE_SURFACE ( 3, 2, ( 
 ( #119298, #237944, #59268 ),
 ( #99696, #241802, #219661 ),
 ( #222214, #120598, #163558 ),
 ( #183132, #21496, #83963 ),
 ( #180557, #181836, #143976 ),
 ( #160995, #240525, #43613 ),
 ( #220942, #22788, #103555 ),
 ( #244360, #246931, #70907 ),
 ( #245661, #107428, #65736 ),
 ( #166161, #167433, #30485 ) ),
 .UNSPECIFIED., .F., .F., .F. ) 
 B_SPLINE_SURFACE_WITH_KNOTS ( ( 4, 2, 2, 2, 4 ),
 ( 3, 3 ),
 ( 0.002161241639767248670, 0.002579950749615824400, 0.002789305304540112482, 0.002893982582002256523, 0.002998659859464400564 ),
 ( 0.000000000000000000, 1.000000000000000000 ),
 .UNSPECIFIED. ) 
 GEOMETRIC_REPRESENTATION_ITEM ( )  RATIONAL_B_SPLINE_SURFACE ( (
 ( 1.000000000000000000, 0.7071067811865475727, 1.000000000000000000),
 ( 1.000000000000000000, 0.7632447400667299320, 1.000000000000000000),
 ( 1.000000000000000000, 0.8158073005105956899, 1.000000000000000000),
 ( 1.000000000000000000, 0.8906973462397930197, 1.000000000000000000),
 ( 1.000000000000000000, 0.9149408947800677927, 1.000000000000000000),
 ( 1.000000000000000000, 0.9493368785275483335, 1.000000000000000000),
 ( 1.000000000000000000, 0.9605194247156682019, 1.000000000000000000),
 ( 1.000000000000000000, 0.9803630264781214576, 1.000000000000000000),
 ( 1.000000000000000000, 0.9900844824271117783, 1.000000000000000000),
 ( 1.000000000000000000, 0.9894588281429294030, 1.000000000000000000) ) ) 
 REPRESENTATION_ITEM ( '' )  SURFACE ( )  );
#239853=ORIENTED_EDGE ( 'NONE', *, *, #139982, .F. ) ;
#239974=EDGE_LOOP ( 'NONE', ( #244036, #127247, #114858, #116152, #9473 ) ) ;
#240092=ORIENTED_EDGE ( 'NONE', *, *, #49360, .T. ) ;
#240340=CARTESIAN_POINT ( 'NONE',  ( 13.99999999999999822, 9.849999999999981881, -16.74999999999999645 ) ) ;
#240439=VECTOR ( 'NONE', #234499, 1000.000000000000000 ) ;
#240522=CARTESIAN_POINT ( 'NONE',  ( -16.80438519320023616, 9.949779096468343909, -12.65073828092127250 ) ) ;
#240525=CARTESIAN_POINT ( 'NONE',  ( -16.85722902420155123, 9.949999999999985079, -20.73445252622950719 ) ) ;
#240544=CARTESIAN_POINT ( 'NONE',  ( -16.94107738177415712, 10.01423928513662176, -12.55000000000000249 ) ) ;
#240819=ADVANCED_FACE ( 'NONE', ( #136300 ), #157211, .F. ) ;
#240909=LINE ( 'NONE', #242178, #139464 ) ;
#240973=AXIS2_PLACEMENT_3D ( 'NONE', #228827, #224942, #108864 ) ;
#240986=EDGE_LOOP ( 'NONE', ( #68478, #196931, #219426, #254363 ) ) ;
#241546=CARTESIAN_POINT ( 'NONE',  ( 16.87683809663749557, 9.949999999999976197, -20.85000000000000142 ) ) ;
#241642=ORIENTED_EDGE ( 'NONE', *, *, #71251, .F. ) ;
#241674=CARTESIAN_POINT ( 'NONE',  ( 22.88900146558018989, 8.703904791112817563, -9.250000000000001776 ) ) ;
#241787=VERTEX_POINT ( 'NONE', #26607 ) ;
#241802=CARTESIAN_POINT ( 'NONE',  ( -16.89155683852570888, 9.949999999999981526, -20.22262815045992923 ) ) ;
#241824=AXIS2_PLACEMENT_3D ( 'NONE', #233915, #55242, #165557 ) ;
#241910=DIRECTION ( 'NONE',  ( 1.073024830501117725E-15, -0.000000000000000000, -1.000000000000000000 ) ) ;
#242126=VECTOR ( 'NONE', #190688, 1000.000000000000000 ) ;
#242178=CARTESIAN_POINT ( 'NONE',  ( -15.55912972643741199, 8.490870273562562076, -12.65000000000000213 ) ) ;
#242260=LINE ( 'NONE', #23258, #101316 ) ;
#242344=FACE_OUTER_BOUND ( 'NONE', #206062, .T. ) ;
#242359=EDGE_LOOP ( 'NONE', ( #44019, #202982, #131599, #219179, #149581 ) ) ;
#242465=FACE_OUTER_BOUND ( 'NONE', #85642, .T. ) ;
#242746=CARTESIAN_POINT ( 'NONE',  ( -14.00000000000000178, 9.849999999999978328, -16.75000000000000355 ) ) ;
#242788=CIRCLE ( 'NONE', #138690, 0.09999999999999939493 ) ;
#242861=CARTESIAN_POINT ( 'NONE',  ( 12.25000000000000000, 9.349999999999983658, -16.74999999999999645 ) ) ;
#242884=CARTESIAN_POINT ( 'NONE',  ( 23.24999999999999645, 11.74999999999998224, -9.250000000000001776 ) ) ;
#242899=LINE ( 'NONE', #5553, #248762 ) ;
#242964=PLANE ( 'NONE',  #6469 ) ;
#243314=ORIENTED_EDGE ( 'NONE', *, *, #127937, .F. ) ;
#243387=CARTESIAN_POINT ( 'NONE',  ( -16.90257928357874917, 9.954106821105362712, -12.63628543011369842 ) ) ;
#243391=EDGE_CURVE ( 'NONE', #206683, #166202, #228635, .T. ) ;
#243543=FACE_OUTER_BOUND ( 'NONE', #147276, .T. ) ;
#243548=CARTESIAN_POINT ( 'NONE',  ( -16.91256925476569606, 9.985731158128174911, -20.96764248900527505 ) ) ;
#243606=ADVANCED_FACE ( 'NONE', ( #80830 ), #156577, .F. ) ;
#243933=CARTESIAN_POINT ( 'NONE',  ( -13.22483237240078324, 9.436674251842845251, -15.17686193099921255 ) ) ;
#243957=LINE ( 'NONE', #10503, #16867 ) ;
#244036=ORIENTED_EDGE ( 'NONE', *, *, #243391, .F. ) ;
#244146=EDGE_LOOP ( 'NONE', ( #181809, #127991, #64947, #200052 ) ) ;
#244267=EDGE_CURVE ( 'NONE', #86390, #67836, #191224, .T. ) ;
#244360=CARTESIAN_POINT ( 'NONE',  ( -16.80621392010911563, 9.942202577507737615, -20.81040803458294164 ) ) ;
#244392=CARTESIAN_POINT ( 'NONE',  ( -18.36973785203556275, 11.47550320048421924, -24.25000000000000000 ) ) ;
#244533=ORIENTED_EDGE ( 'NONE', *, *, #238293, .F. ) ;
#244537=COLOUR_RGB ( '', 0.66274510, 0.83137255, 0.94901961) ;
#244667=DIRECTION ( 'NONE',  ( -1.073024830501117725E-15, 0.000000000000000000, 1.000000000000000000 ) ) ;
#244879=EDGE_CURVE ( 'NONE', #237173, #28990, #222461, .T. ) ;
#244999=CARTESIAN_POINT ( 'NONE',  ( -16.93230518875208190, 10.00075036141984164, -12.57577834810150108 ) ) ;
#245001=DIRECTION ( 'NONE',  ( -0.000000000000000000, -0.000000000000000000, -1.000000000000000000 ) ) ;
#245067=ORIENTED_EDGE ( 'NONE', *, *, #76450, .T. ) ;
#245177=CIRCLE ( 'NONE', #252972, 0.9000000000000014655 ) ;
#245265=CARTESIAN_POINT ( 'NONE',  ( -18.40000000000000213, 11.47316190336248809, -20.94999999999999929 ) ) ;
#245424=EDGE_CURVE ( 'NONE', #146218, #95294, #251116, .T. ) ;
#245473=LINE ( 'NONE', #242884, #27497 ) ;
#245559=ORIENTED_EDGE ( 'NONE', *, *, #189871, .F. ) ;
#245661=CARTESIAN_POINT ( 'NONE',  ( -16.79270642812308978, 9.946244216938064042, -20.83893327856252142 ) ) ;
#245773=CARTESIAN_POINT ( 'NONE',  ( -16.77732147262506146, 9.945966932618629741, -20.83649124327587643 ) ) ;
#245972=CARTESIAN_POINT ( 'NONE',  ( -18.40000000000000213, 11.74999999999998224, -20.85000000000000142 ) ) ;
#245977=DIRECTION ( 'NONE',  ( 1.000000000000000000, 0.000000000000000000, 1.073024830501117725E-15 ) ) ;
#246120=CARTESIAN_POINT ( 'NONE',  ( 18.39999999999997371, 11.47316190336247388, -24.25000000000001066 ) ) ;
#246122=FACE_OUTER_BOUND ( 'NONE', #240986, .T. ) ;
#246128=CARTESIAN_POINT ( 'NONE',  ( -16.92973740335364496, 9.992503814467408318, -20.90605903520226505 ) ) ;
#246196=ORIENTED_EDGE ( 'NONE', *, *, #90030, .T. ) ;
#246203=CARTESIAN_POINT ( 'NONE',  ( -16.89268316805465986, 9.951721813242182080, -20.85575247854553993 ) ) ;
#246505=CARTESIAN_POINT ( 'NONE',  ( -15.70407651835961005, 9.355806591630130953, -16.29110253154617283 ) ) ;
#246736=ORIENTED_EDGE ( 'NONE', *, *, #71525, .F. ) ;
#246870=DIRECTION ( 'NONE',  ( 0.000000000000000000, -1.000000000000000000, 0.000000000000000000 ) ) ;
#246931=CARTESIAN_POINT ( 'NONE',  ( -16.82055514392389028, 9.949999999999983302, -20.82320192545794768 ) ) ;
#246938=PLANE ( 'NONE',  #73843 ) ;
#246974=VECTOR ( 'NONE', #250277, 1000.000000000000000 ) ;
#247480=CARTESIAN_POINT ( 'NONE',  ( -16.87036670365548474, 9.989418819301645769, -20.97956011730205006 ) ) ;
#247500=EDGE_CURVE ( 'NONE', #229697, #181378, #67632, .T. ) ;
#247550=CIRCLE ( 'NONE', #135087, 0.09999999999999939493 ) ;
#247679=VECTOR ( 'NONE', #168439, 1000.000000000000000 ) ;
#247758=EDGE_LOOP ( 'NONE', ( #111251, #177509, #232242, #221630, #84585 ) ) ;
#247928=B_SPLINE_CURVE_WITH_KNOTS ( 'NONE', 3,
 ( #198828, #20208, #219669, #237949, #223515, #44903, #197538, #63160, #21501, #22795, #3180, #202679, #162294, #99701 ),
 .UNSPECIFIED., .F., .F.,
 ( 4, 2, 2, 2, 2, 2, 4 ),
 ( 1.398578778534940505E-17, 0.0003823333598417854922, 0.0005735000397626704863, 0.0006690833797231130918, 0.0007168750497033329850, 0.0007407708846934382696, 0.0007646667196835435542 ),
 .UNSPECIFIED. ) ;
#247943=( GEOMETRIC_REPRESENTATION_CONTEXT ( 3 ) GLOBAL_UNCERTAINTY_ASSIGNED_CONTEXT ( ( #194073 ) ) GLOBAL_UNIT_ASSIGNED_CONTEXT ( ( #236890, #114379, #193931 ) ) REPRESENTATION_CONTEXT ( 'NONE', 'WORKASPACE' ) );
#247973=AXIS2_PLACEMENT_3D ( 'NONE', #177546, #197050, #137095 ) ;
#248039=ORIENTED_EDGE ( 'NONE', *, *, #178791, .F. ) ;
#248097=VERTEX_POINT ( 'NONE', #153319 ) ;
#248116=DIRECTION ( 'NONE',  ( -1.073024830501117725E-15, 0.000000000000000000, 1.000000000000000000 ) ) ;
#248159=( BOUNDED_CURVE ( )  B_SPLINE_CURVE ( 3, ( #51944, #50661, #170688, #152383 ),
 .UNSPECIFIED., .F., .F. ) 
 B_SPLINE_CURVE_WITH_KNOTS ( ( 4, 4 ),
 ( 5.731445031868799056, 5.983100554402348337 ),
 .UNSPECIFIED. ) 
 CURVE ( )  GEOMETRIC_REPRESENTATION_ITEM ( )  RATIONAL_B_SPLINE_CURVE ( ( 1.000000000000000000, 0.9947294176030464508, 0.9947294176030464508, 1.000000000000000000 ) ) 
 REPRESENTATION_ITEM ( '' )  );
#248228=CARTESIAN_POINT ( 'NONE',  ( -16.92280123533711489, 9.949999999999983302, -12.85063231408517659 ) ) ;
#248238=FACE_OUTER_BOUND ( 'NONE', #234959, .T. ) ;
#248335=CARTESIAN_POINT ( 'NONE',  ( -16.77828822459933633, 9.946229375056461208, -20.83737174908105771 ) ) ;
#248392=EDGE_LOOP ( 'NONE', ( #108790, #52201, #197789, #122644 ) ) ;
#248439=ADVANCED_FACE ( 'NONE', ( #150430 ), #28030, .F. ) ;
#248472=CARTESIAN_POINT ( 'NONE',  ( -16.97683809663752186, 9.849999999999983658, -20.09763598180368405 ) ) ;
#248522=CARTESIAN_POINT ( 'NONE',  ( -16.27683809663751191, 9.349999999999976552, -12.55000000000000249 ) ) ;
#248762=VECTOR ( 'NONE', #164662, 1000.000000000000000 ) ;
#248859=CARTESIAN_POINT ( 'NONE',  ( -16.94180778212363236, 9.992443055732147528, -12.60418357053324634 ) ) ;
#248862=LINE ( 'NONE', #89767, #28914 ) ;
#249048=ORIENTED_EDGE ( 'NONE', *, *, #139982, .T. ) ;
#249110=VECTOR ( 'NONE', #87791, 1000.000000000000000 ) ;
#249147=B_SPLINE_CURVE_WITH_KNOTS ( 'NONE', 3,
 ( #67022, #207850, #128290, #226062, #146533, #168747, #126995, #107427, #29224, #108718, #43611, #89143, #4466, #83962, #163557, #170023, #93002, #12209, #13481, #134678, #91722, #190858, #228683, #111292, #90422, #149148, #214243, #210400, #249525, #211690 ),
 .UNSPECIFIED., .F., .F.,
 ( 4, 2, 2, 2, 2, 2, 2, 2, 2, 2, 2, 2, 2, 2, 4 ),
 ( 0.000000000000000000, 0.0003422764154113329101, 0.0006845528308226658202, 0.001026829246233998622, 0.001369105661645331640, 0.002053658492468000713, 0.002738211323290670220, 0.003080487738702004756, 0.003422764154113339726, 0.003765040569524674696, 0.004107316984936008365, 0.004449593400347343769, 0.004791869815758678305, 0.005134146231170012842, 0.005476422646581347378 ),
 .UNSPECIFIED. ) ;
#249261=AXIS2_PLACEMENT_3D ( 'NONE', #15938, #211544, #52443 ) ;
#249460=CARTESIAN_POINT ( 'NONE',  ( -16.93388492042257809, 9.988541822515902169, -20.90054512318617697 ) ) ;
#249522=CARTESIAN_POINT ( 'NONE',  ( -16.97683809663752186, 9.949999999999983302, -13.40236401819648648 ) ) ;
#249525=CARTESIAN_POINT ( 'NONE',  ( 12.25000000000000000, 9.349999999999983658, -16.86426760761609600 ) ) ;
#249614=AXIS2_PLACEMENT_3D ( 'NONE', #177044, #19226, #17932 ) ;
#249623=ORIENTED_EDGE ( 'NONE', *, *, #105908, .F. ) ;
#249794=DIRECTION ( 'NONE',  ( 1.000000000000000000, 1.186688945009009831E-16, 0.000000000000000000 ) ) ;
#249825=DIRECTION ( 'NONE',  ( 1.000000000000000000, 0.000000000000000000, -0.000000000000000000 ) ) ;
#249899=VERTEX_POINT ( 'NONE', #178990 ) ;
#250164=VECTOR ( 'NONE', #40144, 1000.000000000000000 ) ;
#250166=CARTESIAN_POINT ( 'NONE',  ( -15.69373346032659455, 9.356790025045880199, -17.20482650861390539 ) ) ;
#250277=DIRECTION ( 'NONE',  ( 1.186688945009010077E-16, -1.000000000000000000, -0.000000000000000000 ) ) ;
#250309=ORIENTED_EDGE ( 'NONE', *, *, #159260, .T. ) ;
#250444=EDGE_CURVE ( 'NONE', #134996, #222282, #110473, .T. ) ;
#250699=ADVANCED_FACE ( 'NONE', ( #253997 ), #135328, .F. ) ;
#250784=CARTESIAN_POINT ( 'NONE',  ( -16.82055514392378726, 9.949999999999985079, -12.67679807454204344 ) ) ;
#250806=ORIENTED_EDGE ( 'NONE', *, *, #170786, .T. ) ;
#250995=DIRECTION ( 'NONE',  ( 0.000000000000000000, 1.000000000000000000, -0.000000000000000000 ) ) ;
#251116=( BOUNDED_CURVE ( )  B_SPLINE_CURVE ( 3, ( #117021, #115738, #79156, #173198 ),
 .UNSPECIFIED., .F., .F. ) 
 B_SPLINE_CURVE_WITH_KNOTS ( ( 4, 4 ),
 ( 0.000000000000000000, 1.570796326794884346 ),
 .UNSPECIFIED. ) 
 CURVE ( )  GEOMETRIC_REPRESENTATION_ITEM ( )  RATIONAL_B_SPLINE_CURVE ( ( 1.000000000000000000, 0.8047378541243679351, 0.8047378541243679351, 1.000000000000000000 ) ) 
 REPRESENTATION_ITEM ( '' )  );
#251187=DIRECTION ( 'NONE',  ( -0.000000000000000000, -0.000000000000000000, -1.000000000000000000 ) ) ;
#251455=CARTESIAN_POINT ( 'NONE',  ( -16.85939591225058365, 9.905226478387843869, -12.96006824646904931 ) ) ;
#251969=EDGE_CURVE ( 'NONE', #816, #194778, #240909, .T. ) ;
#252008=CARTESIAN_POINT ( 'NONE',  ( -20.65000000000000568, 7.249999999999983125, -12.65000000000000213 ) ) ;
#252071=CARTESIAN_POINT ( 'NONE',  ( -16.82542659449985223, 9.934499891427440943, -12.74463560002616624 ) ) ;
#252287=CARTESIAN_POINT ( 'NONE',  ( 12.29592348164039350, 9.355806591630123847, -16.29110253154616217 ) ) ;
#252313=LINE ( 'NONE', #209346, #36562 ) ;
#252340=CARTESIAN_POINT ( 'NONE',  ( -18.37160782347004329, 11.47561641480238492, -9.250000000000001776 ) ) ;
#252727=CARTESIAN_POINT ( 'NONE',  ( -16.87683809663752399, 9.849999999999988987, -13.40236401819630530 ) ) ;
#252972=AXIS2_PLACEMENT_3D ( 'NONE', #202792, #241910, #141527 ) ;
#253160=ORIENTED_EDGE ( 'NONE', *, *, #209129, .T. ) ;
#253418=DIRECTION ( 'NONE',  ( 1.073024830501117725E-15, -0.000000000000000000, -1.000000000000000000 ) ) ;
#253467=CARTESIAN_POINT ( 'NONE',  ( -16.94107738177415712, 10.01423928513662176, -12.55000000000000249 ) ) ;
#253575=CARTESIAN_POINT ( 'NONE',  ( 13.88302573338718915, 9.457410944767412175, -15.00008397379001934 ) ) ;
#253655=DIRECTION ( 'NONE',  ( -1.000000000000000000, 0.000000000000000000, 0.000000000000000000 ) ) ;
#253959=ADVANCED_FACE ( 'NONE', ( #40603 ), #38023, .F. ) ;
#253997=FACE_OUTER_BOUND ( 'NONE', #242359, .T. ) ;
#254231=B_SPLINE_CURVE_WITH_KNOTS ( 'NONE', 3,
 ( #246203, #88381, #209641, #67559, #111833, #31041, #132680, #28480, #8875, #247480 ),
 .UNSPECIFIED., .F., .F.,
 ( 4, 3, 3, 4 ),
 ( 7.632826238683908479E-06, 4.756916949875909513E-05, 9.484459048150660151E-05, 0.0001435500935099896477 ),
 .UNSPECIFIED. ) ;
#254281=ORIENTED_EDGE ( 'NONE', *, *, #179288, .T. ) ;
#254363=ORIENTED_EDGE ( 'NONE', *, *, #188004, .T. ) ;
#254638=VERTEX_POINT ( 'NONE', #20072 ) ;
#254751=CARTESIAN_POINT ( 'NONE',  ( -16.87368910959167678, 9.961273816691395666, -12.61249309664058948 ) ) ;
#254816=CARTESIAN_POINT ( 'NONE',  ( 12.47034474403012361, 9.375538102048006195, -15.86987588099082735 ) ) ;
#255032=CARTESIAN_POINT ( 'NONE',  ( -16.93521499325732549, 9.994786119803523050, -20.90710854109355310 ) ) ;
#255070=ORIENTED_EDGE ( 'NONE', *, *, #218716, .F. ) ;
#255350=ORIENTED_EDGE ( 'NONE', *, *, #40377, .F. ) ;
#255369=CARTESIAN_POINT ( 'NONE',  ( 18.39999999999997371, 11.74999999999998224, -9.250000000000001776 ) ) ;
#255457=AXIS2_PLACEMENT_3D ( 'NONE', #228135, #43385, #49489 ) ;
#255566=CARTESIAN_POINT ( 'NONE',  ( -16.94225986326250322, 9.949999999999981526, -12.94671937560788599 ) ) ;
#255634=CARTESIAN_POINT ( 'NONE',  ( -18.40000000000000213, 11.48667500175767131, -24.25000000000000000 ) ) ;
#255705=EDGE_CURVE ( 'NONE', #88402, #187424, #254231, .T. ) ;
#255760=ORIENTED_EDGE ( 'NONE', *, *, #48208, .F. ) ;
#255866=DIRECTION ( 'NONE',  ( -1.000000000000000000, 0.000000000000000000, 0.000000000000000000 ) ) ;
#255930=CARTESIAN_POINT ( 'NONE',  ( 15.48841904831874849, 8.561580951681223794, -12.64999999999999858 ) ) ;
#255955=CARTESIAN_POINT ( 'NONE',  ( -23.25000000000000355, 10.04999999999998295, -20.75000000000000000 ) ) ;
#256304=ORIENTED_EDGE ( 'NONE', *, *, #28727, .F. ) ;
#256441=CARTESIAN_POINT ( 'NONE',  ( -18.40000000000000213, 11.33174054712516110, -12.65000000000000213 ) ) ;
#256449=B_SPLINE_CURVE_WITH_KNOTS ( 'NONE', 3,
 ( #175793, #132814, #135345, #212355, #74141, #231917, #235734, #94940, #173261, #213605, #251455, #117090, #214895, #252727 ),
 .UNSPECIFIED., .F., .F.,
 ( 4, 2, 2, 2, 2, 2, 4 ),
 ( 0.000000000000000000, 2.389617747642649214E-05, 4.779235495285298429E-05, 9.558470990571555021E-05, 0.0001911694198114329165, 0.0003823388396228745065, 0.0007646776792457625656 ),
 .UNSPECIFIED. ) ;
#256797=DIRECTION ( 'NONE',  ( -0.000000000000000000, 1.000000000000000000, -0.000000000000000000 ) ) ;
#256868=DIRECTION ( 'NONE',  ( 0.000000000000000000, 0.000000000000000000, -1.000000000000000000 ) ) ;
#256882=CARTESIAN_POINT ( 'NONE',  ( -18.41431012584568805, 11.48747202920816868, -9.226763986898326664 ) ) ;
#257145=CARTESIAN_POINT ( 'NONE',  ( 20.99999999999999645, 9.749999999999982236, -9.250000000000001776 ) ) ;
#257308=CARTESIAN_POINT ( 'NONE',  ( -16.86757978335471719, 9.965650379034281414, -12.59800465316751250 ) ) ;
#257454=FACE_OUTER_BOUND ( 'NONE', #82282, .T. ) ;
#257675=SURFACE_STYLE_FILL_AREA ( #176950 ) ;
#257817=LINE ( 'NONE', #17968, #250164 ) ;
#257864=AXIS2_PLACEMENT_3D ( 'NONE', #145716, #46608, #126151 ) ;
#258053=VERTEX_POINT ( 'NONE', #145742 ) ;
ENDSEC;
END-ISO-10303-21;
